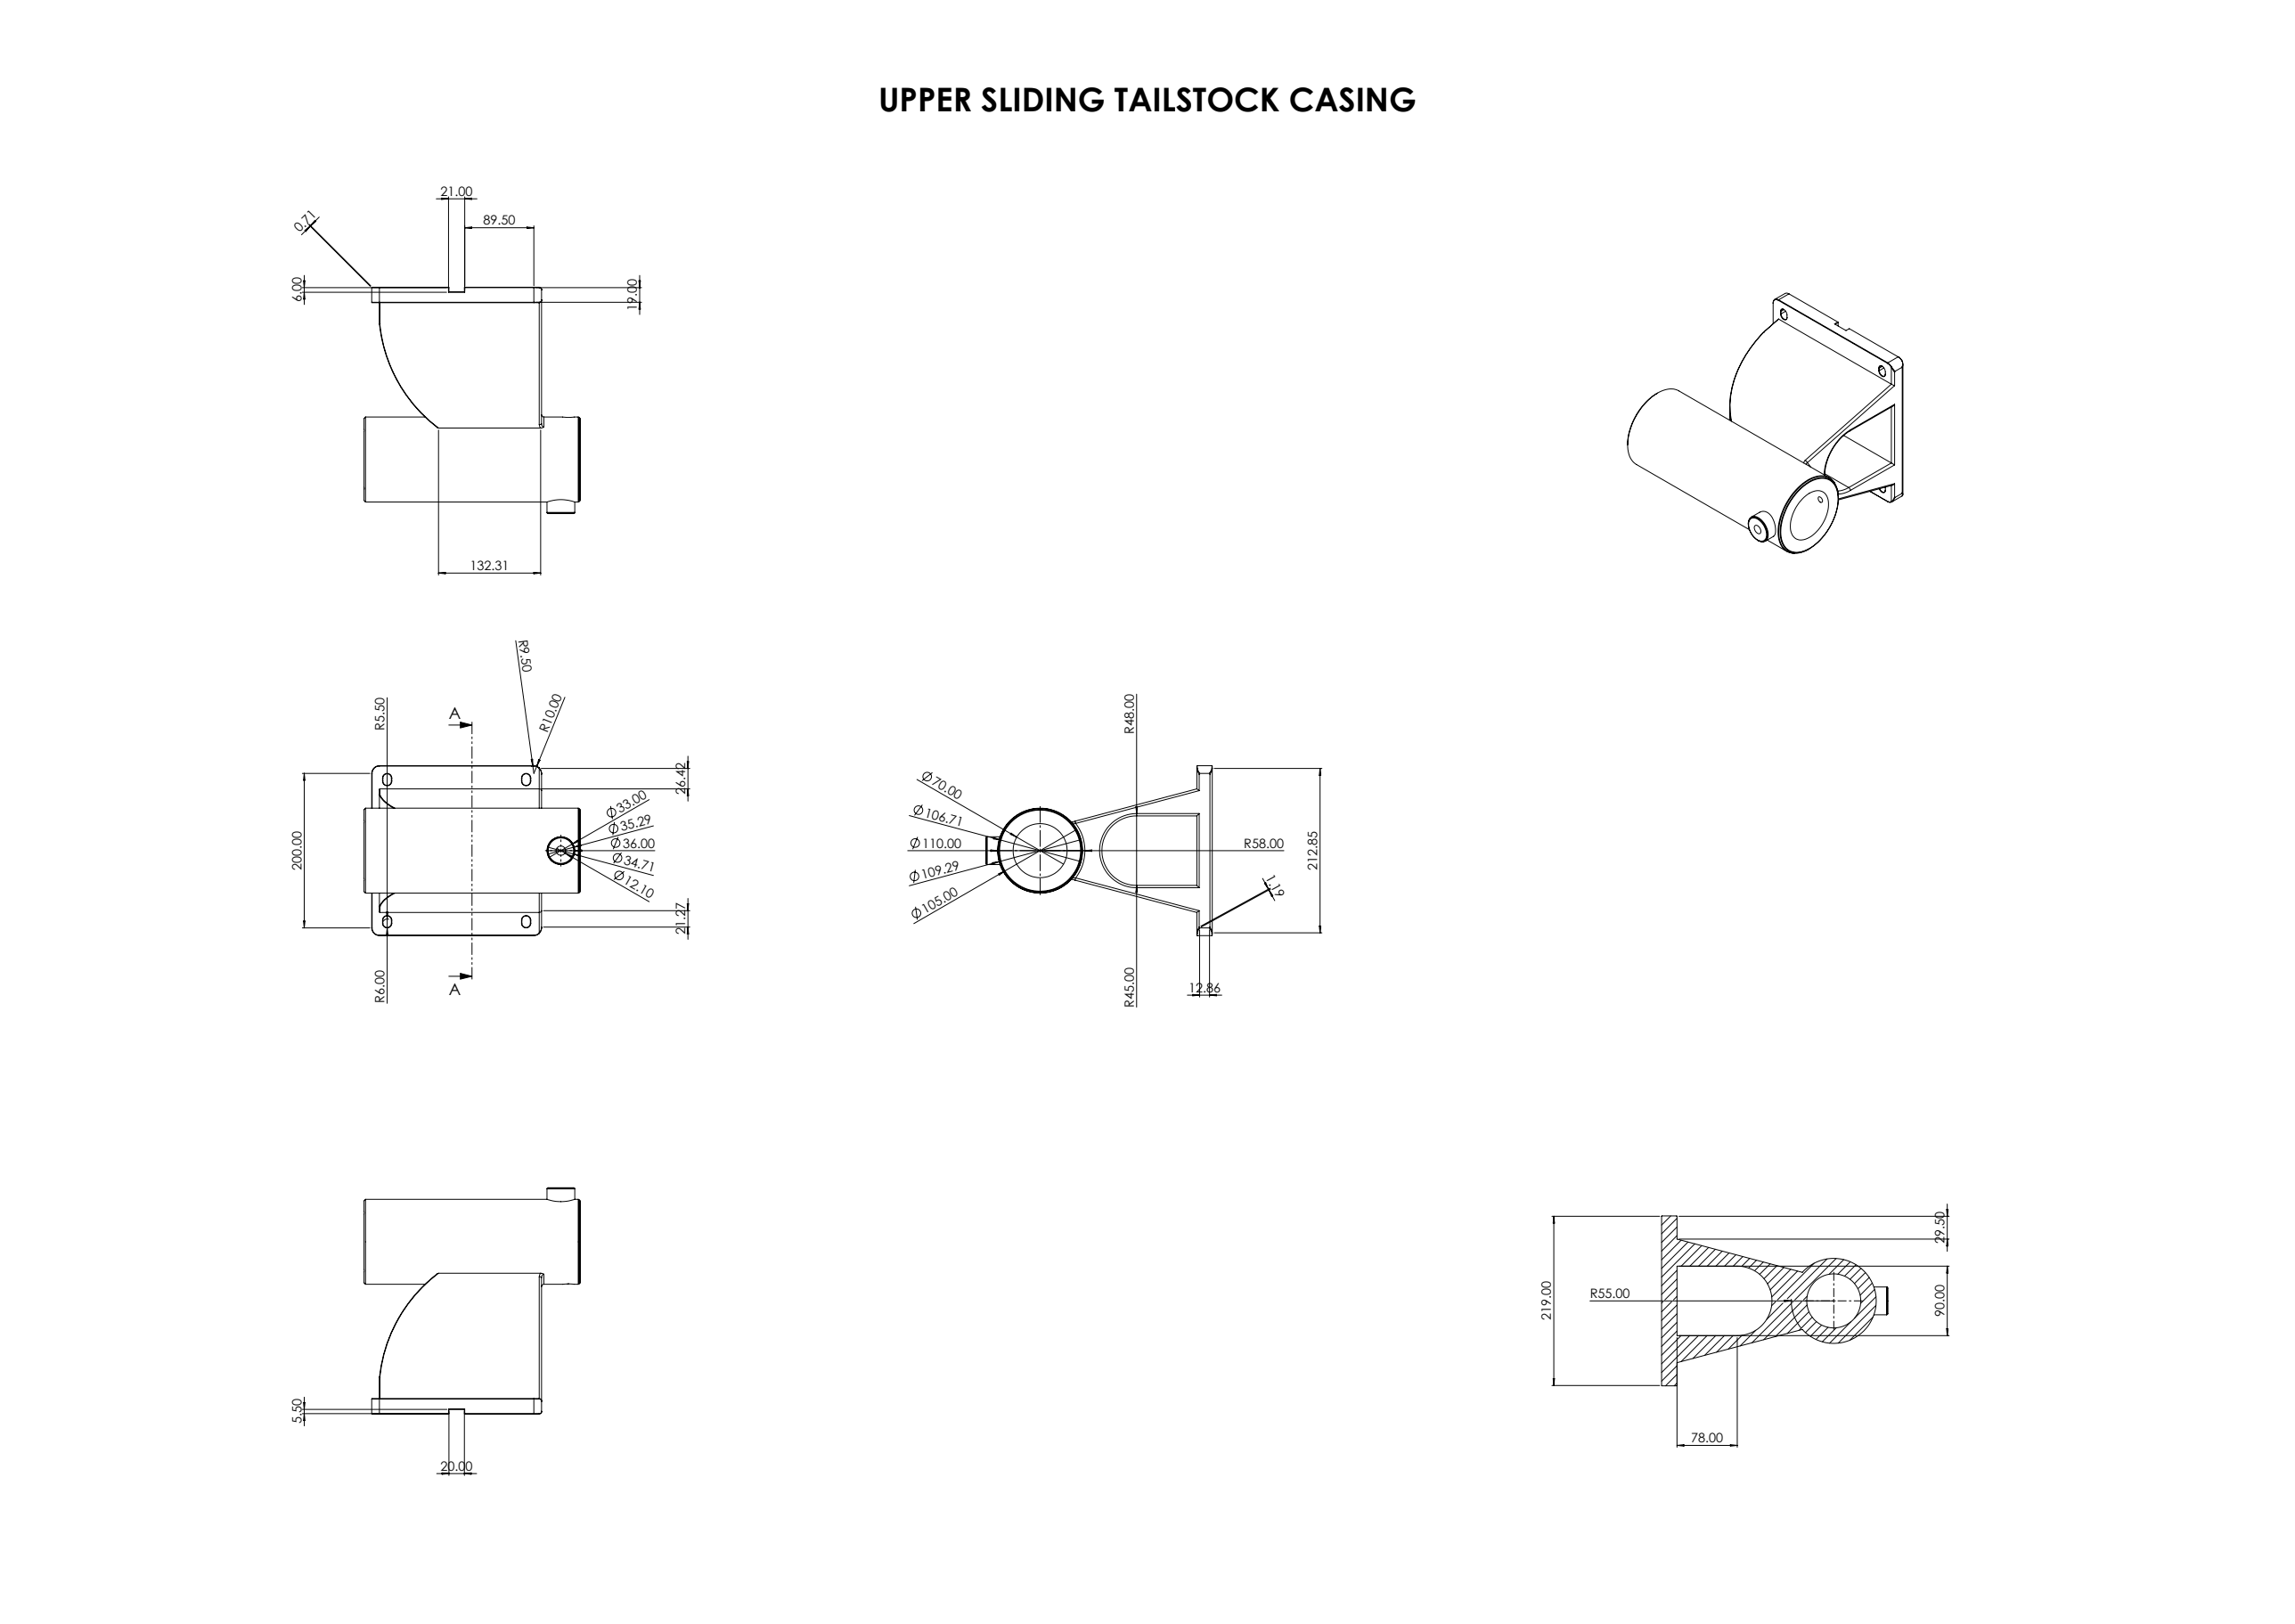
ISO-10303-21;
HEADER;
/* Generated by software containing ST-Developer
 * from STEP Tools, Inc. (www.steptools.com) 
 */

FILE_DESCRIPTION(
/* description */ (''),
/* implementation_level */ '2;1');

FILE_NAME(
/* name */ '02_Upper_Sliding_Tailstock_Casing.step',
/* time_stamp */ '2026-10-26T03:50:32-07:00',
/* author */ (''),
/* organization */ (''),
/* preprocessor_version */ 'ST-DEVELOPER v20.2',
/* originating_system */ 'Autodesk Translation Framework v15.15.0.0',
/* authorisation */ '');

FILE_SCHEMA (('AUTOMOTIVE_DESIGN { 1 0 10303 214 3 1 1 }'));
ENDSEC;

DATA;
#10=MECHANICAL_DESIGN_GEOMETRIC_PRESENTATION_REPRESENTATION('',(#1040),#76660);
#138=B_SPLINE_SURFACE_WITH_KNOTS('',3,3,((#37277,#37278,#37279,#37280,#37281,
#37282,#37283,#37284,#37285,#37286,#37287,#37288,#37289,#37290,#37291,#37292,
#37293,#37294,#37295,#37296,#37297,#37298,#37299,#37300,#37301,#37302,#37303,
#37304,#37305,#37306,#37307,#37308,#37309,#37310,#37311,#37312,#37313,#37314,
#37315,#37316,#37317,#37318,#37319,#37320,#37321,#37322,#37323,#37324),
(#37325,#37326,#37327,#37328,#37329,#37330,#37331,#37332,#37333,#37334,
#37335,#37336,#37337,#37338,#37339,#37340,#37341,#37342,#37343,#37344,#37345,
#37346,#37347,#37348,#37349,#37350,#37351,#37352,#37353,#37354,#37355,#37356,
#37357,#37358,#37359,#37360,#37361,#37362,#37363,#37364,#37365,#37366,#37367,
#37368,#37369,#37370,#37371,#37372),(#37373,#37374,#37375,#37376,#37377,
#37378,#37379,#37380,#37381,#37382,#37383,#37384,#37385,#37386,#37387,#37388,
#37389,#37390,#37391,#37392,#37393,#37394,#37395,#37396,#37397,#37398,#37399,
#37400,#37401,#37402,#37403,#37404,#37405,#37406,#37407,#37408,#37409,#37410,
#37411,#37412,#37413,#37414,#37415,#37416,#37417,#37418,#37419,#37420),
(#37421,#37422,#37423,#37424,#37425,#37426,#37427,#37428,#37429,#37430,
#37431,#37432,#37433,#37434,#37435,#37436,#37437,#37438,#37439,#37440,#37441,
#37442,#37443,#37444,#37445,#37446,#37447,#37448,#37449,#37450,#37451,#37452,
#37453,#37454,#37455,#37456,#37457,#37458,#37459,#37460,#37461,#37462,#37463,
#37464,#37465,#37466,#37467,#37468)),.UNSPECIFIED.,.F.,.T.,.F.,(4,4),(4,
1,1,1,1,1,1,1,1,1,1,1,1,1,1,1,1,1,1,1,1,1,1,1,1,1,1,1,1,1,1,1,1,1,1,1,1,
1,1,1,1,1,1,1,1,4),(0.,1.),(0.,0.301700924572155,0.452551386858232,0.60340184914431,
0.62225815693007,0.641114464715829,0.678827080287349,0.716539695858868,
0.754252311430387,0.829677542573426,0.867390158144946,0.905102773716465,
1.20680369828862,1.23194544200297,1.25708718571731,1.307370673146,1.40793764800339,
1.81020554743293,1.83534729114728,1.86048903486162,1.91077252229031,2.0113394971477,
2.21247344686247,2.26275693429116,2.41360739657724,2.56445785886332,2.71530832114939,
2.86615878343547,2.94158401457851,2.96044032236427,2.97929663015003,2.99815293793579,
3.00758109182867,3.01229516877511,3.01700924572155,3.3187101702937,3.35642278586522,
3.39413540143674,3.46956063257978,3.54498586372282,3.58269847929434,3.6015547870801,
3.62041109486586,3.77126155715194,3.92211201943801,4.22381294401017),
 .UNSPECIFIED.);
#139=B_SPLINE_SURFACE_WITH_KNOTS('',3,3,((#37678,#37679,#37680,#37681,#37682,
#37683,#37684,#37685),(#37686,#37687,#37688,#37689,#37690,#37691,#37692,
#37693),(#37694,#37695,#37696,#37697,#37698,#37699,#37700,#37701),(#37702,
#37703,#37704,#37705,#37706,#37707,#37708,#37709)),.UNSPECIFIED.,.F.,.F.,
 .F.,(4,4),(4,1,1,1,1,4),(0.,1.),(0.,0.142857142857143,0.428571428571429,
0.571428571428571,0.857142857142857,1.),.UNSPECIFIED.);
#140=B_SPLINE_SURFACE_WITH_KNOTS('',3,3,((#37811,#37812,#37813,#37814,#37815,
#37816,#37817,#37818),(#37819,#37820,#37821,#37822,#37823,#37824,#37825,
#37826),(#37827,#37828,#37829,#37830,#37831,#37832,#37833,#37834),(#37835,
#37836,#37837,#37838,#37839,#37840,#37841,#37842)),.UNSPECIFIED.,.F.,.F.,
 .F.,(4,4),(4,1,1,1,1,4),(0.,1.),(0.,0.142857142857143,0.428571428571429,
0.571428571428571,0.857142857142857,1.),.UNSPECIFIED.);
#141=B_SPLINE_SURFACE_WITH_KNOTS('',3,3,((#37944,#37945,#37946,#37947,#37948),
(#37949,#37950,#37951,#37952,#37953),(#37954,#37955,#37956,#37957,#37958),
(#37959,#37960,#37961,#37962,#37963)),.UNSPECIFIED.,.F.,.F.,.F.,(4,4),(4,
1,4),(0.,1.),(1.87779361595245,2.32640602317479,2.66286532859155),
 .UNSPECIFIED.);
#142=B_SPLINE_SURFACE_WITH_KNOTS('',3,3,((#38058,#38059,#38060,#38061),
(#38062,#38063,#38064,#38065),(#38066,#38067,#38068,#38069),(#38070,#38071,
#38072,#38073)),.UNSPECIFIED.,.F.,.F.,.F.,(4,4),(4,4),(0.,1.),(-1.87779361595245,
-1.82480525135948),.UNSPECIFIED.);
#143=B_SPLINE_SURFACE_WITH_KNOTS('',3,3,((#38078,#38079,#38080,#38081,#38082),
(#38083,#38084,#38085,#38086,#38087),(#38088,#38089,#38090,#38091,#38092),
(#38093,#38094,#38095,#38096,#38097)),.UNSPECIFIED.,.F.,.F.,.F.,(4,4),(4,
1,4),(0.,1.),(0.000100035134689748,0.3365592783323,0.78517160259578),
 .UNSPECIFIED.);
#144=B_SPLINE_SURFACE_WITH_KNOTS('',3,3,((#38110,#38111,#38112,#38113),
(#38114,#38115,#38116,#38117),(#38118,#38119,#38120,#38121),(#38122,#38123,
#38124,#38125)),.UNSPECIFIED.,.F.,.F.,.F.,(4,4),(4,4),(0.,1.),(-0.838159967188763,
-0.78517160259578),.UNSPECIFIED.);
#145=B_SPLINE_SURFACE_WITH_KNOTS('',3,3,((#38503,#38504,#38505,#38506,#38507,
#38508,#38509,#38510),(#38511,#38512,#38513,#38514,#38515,#38516,#38517,
#38518),(#38519,#38520,#38521,#38522,#38523,#38524,#38525,#38526),(#38527,
#38528,#38529,#38530,#38531,#38532,#38533,#38534)),.UNSPECIFIED.,.F.,.F.,
 .F.,(4,4),(4,1,1,1,1,4),(0.,1.),(0.,0.142857142857143,0.428571428571429,
0.571428571428571,0.857142857142857,1.),.UNSPECIFIED.);
#146=B_SPLINE_SURFACE_WITH_KNOTS('',3,3,((#38592,#38593,#38594,#38595,#38596,
#38597,#38598,#38599),(#38600,#38601,#38602,#38603,#38604,#38605,#38606,
#38607),(#38608,#38609,#38610,#38611,#38612,#38613,#38614,#38615),(#38616,
#38617,#38618,#38619,#38620,#38621,#38622,#38623)),.UNSPECIFIED.,.F.,.F.,
 .F.,(4,4),(4,1,1,1,1,4),(0.,1.),(0.,0.142857142857143,0.428571428571429,
0.571428571428571,0.857142857142857,1.),.UNSPECIFIED.);
#147=B_SPLINE_SURFACE_WITH_KNOTS('',3,3,((#38722,#38723,#38724,#38725,#38726,
#38727,#38728),(#38729,#38730,#38731,#38732,#38733,#38734,#38735),(#38736,
#38737,#38738,#38739,#38740,#38741,#38742),(#38743,#38744,#38745,#38746,
#38747,#38748,#38749)),.UNSPECIFIED.,.F.,.F.,.F.,(4,4),(4,1,1,1,4),(0.,
1.),(9.97415695384386E-5,0.217192720402113,0.325739209818401,0.542832188650975,
0.75992516748355),.UNSPECIFIED.);
#148=B_SPLINE_SURFACE_WITH_KNOTS('',3,3,((#38791,#38792,#38793,#38794),
(#38795,#38796,#38797,#38798),(#38799,#38800,#38801,#38802),(#38803,#38804,
#38805,#38806)),.UNSPECIFIED.,.F.,.F.,.F.,(4,4),(4,4),(0.,1.),(0.759925167483548,
0.811761172549836),.UNSPECIFIED.);
#149=B_SPLINE_SURFACE_WITH_KNOTS('',3,3,((#38811,#38812,#38813,#38814,#38815,
#38816,#38817,#38818,#38819,#38820),(#38821,#38822,#38823,#38824,#38825,
#38826,#38827,#38828,#38829,#38830),(#38831,#38832,#38833,#38834,#38835,
#38836,#38837,#38838,#38839,#38840),(#38841,#38842,#38843,#38844,#38845,
#38846,#38847,#38848,#38849,#38850)),.UNSPECIFIED.,.F.,.F.,.F.,(4,4),(4,
2,1,1,2,4),(0.,1.),(1.90304005106469,2.0340806772701,2.19643291178007,2.27760902903505,
2.43996126354502,2.66286552223545),.UNSPECIFIED.);
#150=B_SPLINE_SURFACE_WITH_KNOTS('',3,3,((#38862,#38863,#38864,#38865),
(#38866,#38867,#38868,#38869),(#38870,#38871,#38872,#38873),(#38874,#38875,
#38876,#38877)),.UNSPECIFIED.,.F.,.F.,.F.,(4,4),(4,4),(0.,1.),(1.85120404599841,
1.90304005106469),.UNSPECIFIED.);
#151=B_SPLINE_SURFACE_WITH_KNOTS('',3,3,((#38903,#38904,#38905,#38906,#38907,
#38908,#38909,#38910,#38911,#38912,#38913,#38914,#38915,#38916,#38917,#38918,
#38919,#38920,#38921,#38922),(#38923,#38924,#38925,#38926,#38927,#38928,
#38929,#38930,#38931,#38932,#38933,#38934,#38935,#38936,#38937,#38938,#38939,
#38940,#38941,#38942),(#38943,#38944,#38945,#38946,#38947,#38948,#38949,
#38950,#38951,#38952,#38953,#38954,#38955,#38956,#38957,#38958,#38959,#38960,
#38961,#38962),(#38963,#38964,#38965,#38966,#38967,#38968,#38969,#38970,
#38971,#38972,#38973,#38974,#38975,#38976,#38977,#38978,#38979,#38980,#38981,
#38982)),.UNSPECIFIED.,.F.,.F.,.F.,(4,4),(4,1,1,1,1,1,1,1,1,1,1,1,1,1,1,
1,1,4),(0.,1.),(6.93617595249389,7.96866100733354,9.0011460621732,10.0336311170129,
10.5498736444327,11.0661161718525,12.0986012266922,13.1310862815318,13.8194096514249,
14.507733021318,15.1960563912111,16.5727031309973,17.2610265008905,17.7772690283103,
18.2935115557301,19.3259966105698,20.3584816654094,21.3909667202491),
 .UNSPECIFIED.);
#152=B_SPLINE_SURFACE_WITH_KNOTS('',3,3,((#39029,#39030,#39031,#39032),
(#39033,#39034,#39035,#39036),(#39037,#39038,#39039,#39040),(#39041,#39042,
#39043,#39044)),.UNSPECIFIED.,.F.,.F.,.F.,(4,4),(4,4),(0.,1.),(6.91671820418794,
6.93617595249389),.UNSPECIFIED.);
#153=B_SPLINE_SURFACE_WITH_KNOTS('',3,3,((#39053,#39054,#39055,#39056),
(#39057,#39058,#39059,#39060),(#39061,#39062,#39063,#39064),(#39065,#39066,
#39067,#39068)),.UNSPECIFIED.,.F.,.F.,.F.,(4,4),(4,4),(0.,1.),(21.3909667202491,
21.410424468555),.UNSPECIFIED.);
#154=B_SPLINE_SURFACE_WITH_KNOTS('',3,3,((#39101,#39102,#39103,#39104,#39105,
#39106,#39107),(#39108,#39109,#39110,#39111,#39112,#39113,#39114),(#39115,
#39116,#39117,#39118,#39119,#39120,#39121),(#39122,#39123,#39124,#39125,
#39126,#39127,#39128)),.UNSPECIFIED.,.F.,.F.,.F.,(4,4),(4,1,1,1,4),(0.,
1.),(0.645522939086389,0.821861702311259,0.998200465536129,1.23331881650262,
1.46843716746911),.UNSPECIFIED.);
#155=B_SPLINE_SURFACE_WITH_KNOTS('',3,3,((#39165,#39166,#39167,#39168,#39169,
#39170,#39171),(#39172,#39173,#39174,#39175,#39176,#39177,#39178),(#39179,
#39180,#39181,#39182,#39183,#39184,#39185),(#39186,#39187,#39188,#39189,
#39190,#39191,#39192)),.UNSPECIFIED.,.F.,.F.,.F.,(4,4),(4,1,1,1,4),(0.,
1.),(-1.46843716746912,-1.29209840424425,-1.11575964101938,-0.880641290052883,
-0.645522939086389),.UNSPECIFIED.);
#156=B_SPLINE_SURFACE_WITH_KNOTS('',3,3,((#39211,#39212,#39213,#39214,#39215,
#39216),(#39217,#39218,#39219,#39220,#39221,#39222),(#39223,#39224,#39225,
#39226,#39227,#39228),(#39229,#39230,#39231,#39232,#39233,#39234),(#39235,
#39236,#39237,#39238,#39239,#39240)),.UNSPECIFIED.,.F.,.F.,.F.,(4,1,4),
(4,1,1,4),(0.,0.571428571428571,1.),(3.93038111840777,4.35323723299001,
4.63514130937817,4.91704538576632),.UNSPECIFIED.);
#157=B_SPLINE_SURFACE_WITH_KNOTS('',3,3,((#39269,#39270,#39271,#39272,#39273,
#39274),(#39275,#39276,#39277,#39278,#39279,#39280),(#39281,#39282,#39283,
#39284,#39285,#39286),(#39287,#39288,#39289,#39290,#39291,#39292),(#39293,
#39294,#39295,#39296,#39297,#39298)),.UNSPECIFIED.,.F.,.F.,.F.,(4,1,4),
(4,1,1,4),(0.,0.571428571428571,1.),(0.317698823900363,0.599602900914624,
0.740554939421754,1.30436309345028),.UNSPECIFIED.);
#174=B_SPLINE_CURVE_WITH_KNOTS('',3,(#37067,#37068,#37069,#37070,#37071,
#37072,#37073,#37074,#37075,#37076,#37077,#37078,#37079,#37080,#37081,#37082,
#37083,#37084),.UNSPECIFIED.,.F.,.F.,(4,2,2,2,2,2,2,2,4),(0.,0.341830025609023,
0.683660051218047,1.02549007682707,1.36732010243609,1.7090034027405,2.05068670304491,
2.39237000334931,2.73405330365372),.UNSPECIFIED.);
#175=B_SPLINE_CURVE_WITH_KNOTS('',3,(#37085,#37086,#37087,#37088,#37089,
#37090,#37091,#37092,#37093,#37094,#37095,#37096,#37097,#37098,#37099,#37100,
#37101,#37102,#37103,#37104,#37105,#37106,#37107,#37108,#37109,#37110,#37111,
#37112,#37113,#37114,#37115,#37116,#37117,#37118,#37119,#37120,#37121,#37122,
#37123,#37124,#37125,#37126,#37127,#37128,#37129,#37130,#37131,#37132,#37133,
#37134),.UNSPECIFIED.,.F.,.F.,(4,2,2,2,2,2,2,2,2,2,2,2,2,2,2,2,2,2,2,2,
2,2,2,2,4),(2.73405330365372,3.07573660395812,3.41741990426253,3.75910320456694,
4.10078650487134,4.44261653048037,4.78444655608939,5.12627658169841,5.46810660730744,
5.80993663291646,6.15176665852548,6.49359668413451,6.83542670974353,7.17711001004794,
7.51879331035234,7.86047661065675,8.20215991096115,8.54384321126556,8.88552651156997,
9.22720981187437,9.56889311217878,9.9107231377878,10.2525531633968,10.5943831890058,
10.9362132146149),.UNSPECIFIED.);
#176=B_SPLINE_CURVE_WITH_KNOTS('',3,(#37138,#37139,#37140,#37141,#37142,
#37143),.UNSPECIFIED.,.F.,.F.,(4,2,4),(1.71566353344894,1.90989804259815,
2.10413255174736),.UNSPECIFIED.);
#177=B_SPLINE_CURVE_WITH_KNOTS('',3,(#37163,#37164,#37165,#37166,#37167,
#37168),.UNSPECIFIED.,.F.,.F.,(4,2,4),(1.71566348905116,1.90989799807537,
2.10413250709959),.UNSPECIFIED.);
#178=B_SPLINE_CURVE_WITH_KNOTS('',3,(#37172,#37173,#37174,#37175,#37176,
#37177),.UNSPECIFIED.,.F.,.F.,(4,2,4),(1.71529227392093,1.90952573777923,
2.10375920163752),.UNSPECIFIED.);
#179=B_SPLINE_CURVE_WITH_KNOTS('',3,(#37181,#37182,#37183,#37184,#37185,
#37186),.UNSPECIFIED.,.F.,.F.,(4,2,4),(1.7156635334436,1.90989804259278,
2.10413255174196),.UNSPECIFIED.);
#180=B_SPLINE_CURVE_WITH_KNOTS('',3,(#37222,#37223,#37224,#37225),
 .UNSPECIFIED.,.F.,.F.,(4,4),(-1.87779361595245,-1.82480525135948),
 .UNSPECIFIED.);
#181=B_SPLINE_CURVE_WITH_KNOTS('',3,(#37229,#37230,#37231,#37232),
 .UNSPECIFIED.,.F.,.F.,(4,4),(-0.838159967188763,-0.78517160259578),
 .UNSPECIFIED.);
#182=B_SPLINE_CURVE_WITH_KNOTS('',3,(#37473,#37474,#37475,#37476,#37477,
#37478,#37479,#37480,#37481,#37482,#37483,#37484,#37485,#37486,#37487,#37488,
#37489,#37490,#37491,#37492,#37493,#37494,#37495,#37496,#37497,#37498,#37499,
#37500,#37501,#37502,#37503,#37504,#37505,#37506,#37507,#37508,#37509,#37510),
 .UNSPECIFIED.,.F.,.F.,(4,1,1,1,1,1,1,1,1,1,1,1,1,1,1,1,1,1,1,1,1,1,1,1,
1,1,1,1,1,1,1,1,1,1,1,4),(0.,0.301700924572155,0.452551386858232,0.60340184914431,
0.62225815693007,0.641114464715829,0.678827080287349,0.716539695858868,
0.754252311430387,0.829677542573426,0.867390158144946,0.905102773716465,
1.20680369828862,1.23194544200297,1.25708718571731,1.307370673146,1.40793764800339,
1.81020554743293,1.83534729114728,1.86048903486162,1.91077252229031,2.0113394971477,
2.21247344686247,2.26275693429116,2.41360739657724,2.56445785886332,2.71530832114939,
2.86615878343547,2.94158401457851,2.96044032236427,2.97929663015003,2.99815293793579,
3.00758109182867,3.01229516877511,3.01700924572155,3.16785970800763),
 .UNSPECIFIED.);
#183=B_SPLINE_CURVE_WITH_KNOTS('',3,(#37511,#37512,#37513,#37514,#37515,
#37516,#37517,#37518,#37519,#37520,#37521,#37522,#37523,#37524),
 .UNSPECIFIED.,.F.,.F.,(4,1,1,1,1,1,1,1,1,1,1,4),(3.16785970800763,3.3187101702937,
3.35642278586522,3.39413540143674,3.46956063257978,3.54498586372282,3.58269847929434,
3.6015547870801,3.62041109486586,3.77126155715194,3.92211201943801,4.22381294401017),
 .UNSPECIFIED.);
#184=B_SPLINE_CURVE_WITH_KNOTS('',3,(#37525,#37526,#37527,#37528,#37529,
#37530,#37531,#37532,#37533,#37534,#37535,#37536,#37537,#37538,#37539,#37540,
#37541,#37542,#37543,#37544,#37545,#37546,#37547,#37548,#37549,#37550,#37551,
#37552,#37553,#37554,#37555,#37556,#37557,#37558,#37559,#37560,#37561,#37562,
#37563,#37564,#37565,#37566,#37567,#37568,#37569,#37570,#37571,#37572),
 .UNSPECIFIED.,.T.,.F.,(4,1,1,1,1,1,1,1,1,1,1,1,1,1,1,1,1,1,1,1,1,1,1,1,
1,1,1,1,1,1,1,1,1,1,1,1,1,1,1,1,1,1,1,1,1,4),(-4.22381294401017,-3.92211201943801,
-3.77126155715194,-3.62041109486586,-3.6015547870801,-3.58269847929434,
-3.54498586372282,-3.46956063257978,-3.39413540143674,-3.35642278586522,
-3.3187101702937,-3.01700924572155,-3.01229516877511,-3.00758109182867,
-2.99815293793579,-2.97929663015003,-2.96044032236427,-2.94158401457851,
-2.86615878343547,-2.71530832114939,-2.56445785886332,-2.41360739657724,
-2.26275693429116,-2.21247344686247,-2.0113394971477,-1.91077252229031,
-1.86048903486162,-1.83534729114728,-1.81020554743293,-1.40793764800339,
-1.307370673146,-1.25708718571731,-1.23194544200297,-1.20680369828862,-0.905102773716465,
-0.867390158144946,-0.829677542573426,-0.754252311430387,-0.716539695858868,
-0.678827080287349,-0.641114464715829,-0.62225815693007,-0.60340184914431,
-0.452551386858232,-0.301700924572155,0.),.UNSPECIFIED.);
#185=B_SPLINE_CURVE_WITH_KNOTS('',3,(#37583,#37584,#37585,#37586,#37587,
#37588,#37589),.UNSPECIFIED.,.F.,.F.,(4,3,4),(0.,0.0706076080518625,0.140717785645037),
 .UNSPECIFIED.);
#186=B_SPLINE_CURVE_WITH_KNOTS('',3,(#37591,#37592,#37593,#37594,#37595,
#37596,#37597,#37598,#37599,#37600,#37601,#37602,#37603,#37604,#37605,#37606,
#37607,#37608,#37609,#37610,#37611,#37612,#37613,#37614,#37615,#37616,#37617),
 .UNSPECIFIED.,.F.,.F.,(4,2,2,2,2,2,3,2,2,2,2,2,4),(-4.20812861828807,-3.99425066999856,
-3.16073871853832,-2.37055403890373,-1.58036935926916,-0.790184679634578,
0.,0.79018467963458,1.58036935926916,2.37055403890374,3.16073871853832,
3.99425066999856,4.20812861828807),.UNSPECIFIED.);
#187=B_SPLINE_CURVE_WITH_KNOTS('',3,(#37619,#37620,#37621,#37622,#37623,
#37624,#37625),.UNSPECIFIED.,.F.,.F.,(4,3,4),(0.,0.0701050024887815,0.140717775218191),
 .UNSPECIFIED.);
#188=B_SPLINE_CURVE_WITH_KNOTS('',3,(#37629,#37630,#37631,#37632,#37633,
#37634,#37635,#37636,#37637,#37638),.UNSPECIFIED.,.F.,.F.,(4,2,2,2,4),(0.,
0.120853732558559,0.299961593709033,0.490853831409324,0.492261507196457),
 .UNSPECIFIED.);
#189=B_SPLINE_CURVE_WITH_KNOTS('',3,(#37641,#37642,#37643,#37644,#37645,
#37646,#37647,#37648,#37649,#37650),.UNSPECIFIED.,.F.,.F.,(4,2,2,2,4),(-0.00109523829507863,
0.,0.141893095426123,0.28665904951154,0.476004129030812),.UNSPECIFIED.);
#190=B_SPLINE_CURVE_WITH_KNOTS('',3,(#37712,#37713,#37714,#37715,#37716,
#37717,#37718,#37719,#37720,#37721,#37722,#37723,#37724,#37725,#37726,#37727,
#37728,#37729,#37730,#37731,#37732,#37733,#37734,#37735,#37736,#37737,#37738,
#37739,#37740,#37741,#37742,#37743,#37744,#37745,#37746,#37747,#37748,#37749,
#37750,#37751),.UNSPECIFIED.,.F.,.F.,(4,3,3,3,3,3,3,3,3,3,3,3,3,4),(0.,
0.0642058267314402,0.135298039610793,0.216720613163576,0.322214526794598,
0.406937710945273,0.476869411739625,0.550300205763178,0.627974002306146,
0.731399879303705,0.815726896068677,0.88866362574166,0.953773893187292,
1.),.UNSPECIFIED.);
#191=B_SPLINE_CURVE_WITH_KNOTS('',3,(#37753,#37754,#37755,#37756),
 .UNSPECIFIED.,.F.,.F.,(4,4),(0.,1.),.UNSPECIFIED.);
#192=B_SPLINE_CURVE_WITH_KNOTS('',3,(#37758,#37759,#37760,#37761,#37762,
#37763,#37764,#37765,#37766,#37767,#37768,#37769,#37770,#37771,#37772,#37773,
#37774,#37775,#37776,#37777,#37778,#37779,#37780,#37781,#37782,#37783,#37784,
#37785,#37786,#37787,#37788,#37789,#37790,#37791,#37792,#37793,#37794,#37795,
#37796,#37797,#37798,#37799,#37800,#37801,#37802,#37803,#37804,#37805,#37806,
#37807,#37808,#37809),.UNSPECIFIED.,.F.,.F.,(4,3,3,3,3,3,3,3,3,3,3,3,3,
3,3,3,3,4),(0.,0.0470013637169586,0.0964181016740628,0.149229530335118,
0.208169836206556,0.286934368114381,0.357340819180099,0.414362060111408,
0.466217667030896,0.532940458652034,0.585846875133388,0.644811876239638,
0.72711087277581,0.795333154581857,0.850882587463839,0.902663377962928,
0.951331688981464,1.),.UNSPECIFIED.);
#193=B_SPLINE_CURVE_WITH_KNOTS('',3,(#37845,#37846,#37847,#37848,#37849,
#37850,#37851,#37852,#37853,#37854,#37855,#37856,#37857,#37858,#37859,#37860,
#37861,#37862,#37863,#37864,#37865,#37866,#37867,#37868,#37869,#37870,#37871,
#37872,#37873,#37874,#37875,#37876,#37877,#37878,#37879,#37880,#37881,#37882,
#37883,#37884,#37885,#37886,#37887,#37888,#37889,#37890,#37891,#37892,#37893,
#37894,#37895,#37896),.UNSPECIFIED.,.F.,.F.,(4,3,3,3,3,3,3,3,3,3,3,3,3,
3,3,3,3,4),(0.,0.0469954003122149,0.0964054107400102,0.149208793967372,
0.208136804390094,0.286850662832856,0.357279255948468,0.414301991680454,
0.466156507957792,0.532886944463068,0.585793820692173,0.644755325044784,
0.727049300721868,0.795286975541401,0.85084796357777,0.9026376409811,0.95131882049055,
1.),.UNSPECIFIED.);
#194=B_SPLINE_CURVE_WITH_KNOTS('',3,(#37898,#37899,#37900,#37901),
 .UNSPECIFIED.,.F.,.F.,(4,4),(-1.,0.),.UNSPECIFIED.);
#195=B_SPLINE_CURVE_WITH_KNOTS('',3,(#37903,#37904,#37905,#37906,#37907,
#37908,#37909,#37910,#37911,#37912,#37913,#37914,#37915,#37916,#37917,#37918,
#37919,#37920,#37921,#37922,#37923,#37924,#37925,#37926,#37927,#37928,#37929,
#37930,#37931,#37932,#37933,#37934,#37935,#37936,#37937,#37938,#37939,#37940,
#37941,#37942),.UNSPECIFIED.,.F.,.F.,(4,3,3,3,3,3,3,3,3,3,3,3,3,4),(0.,
0.0642045803508197,0.135295214744166,0.216715461741643,0.322211745001425,
0.406935276876247,0.476866299954066,0.550298370624421,0.62797200200528,
0.73139484549015,0.815724459936111,0.888662483366991,0.953773603714735,
1.),.UNSPECIFIED.);
#196=B_SPLINE_CURVE_WITH_KNOTS('',3,(#37964,#37965,#37966,#37967,#37968),
 .UNSPECIFIED.,.F.,.F.,(4,1,4),(-2.66286532859155,-2.32640602317479,-1.87779361595245),
 .UNSPECIFIED.);
#197=B_SPLINE_CURVE_WITH_KNOTS('',3,(#37971,#37972,#37973,#37974,#37975),
 .UNSPECIFIED.,.F.,.F.,(4,1,4),(1.87779361595245,2.32640602317479,2.66286532859155),
 .UNSPECIFIED.);
#198=B_SPLINE_CURVE_WITH_KNOTS('',3,(#38074,#38075,#38076,#38077),
 .UNSPECIFIED.,.F.,.F.,(4,4),(1.82480525135948,1.87779361595245),
 .UNSPECIFIED.);
#199=B_SPLINE_CURVE_WITH_KNOTS('',3,(#38099,#38100,#38101,#38102,#38103),
 .UNSPECIFIED.,.F.,.F.,(4,1,4),(0.000100035134689748,0.3365592783323,0.78517160259578),
 .UNSPECIFIED.);
#200=B_SPLINE_CURVE_WITH_KNOTS('',3,(#38105,#38106,#38107,#38108,#38109),
 .UNSPECIFIED.,.F.,.F.,(4,1,4),(-0.78517160259578,-0.3365592783323,-0.000100035134689748),
 .UNSPECIFIED.);
#201=B_SPLINE_CURVE_WITH_KNOTS('',3,(#38126,#38127,#38128,#38129),
 .UNSPECIFIED.,.F.,.F.,(4,4),(0.78517160259578,0.838159967188763),
 .UNSPECIFIED.);
#202=B_SPLINE_CURVE_WITH_KNOTS('',3,(#38140,#38141,#38142,#38143,#38144,
#38145,#38146,#38147,#38148,#38149,#38150,#38151,#38152,#38153,#38154,#38155,
#38156,#38157,#38158,#38159,#38160,#38161,#38162,#38163,#38164,#38165,#38166,
#38167,#38168,#38169,#38170,#38171,#38172,#38173,#38174,#38175,#38176,#38177,
#38178,#38179),.UNSPECIFIED.,.F.,.F.,(4,3,3,3,3,3,3,3,3,3,3,3,3,4),(0.,
0.0642049615968745,0.13529611806662,0.216717311062181,0.322210830481009,
0.406934476670883,0.476865564838168,0.550296903893395,0.627969426873969,
0.73138741425766,0.815717741324156,0.888655709551853,0.95376643384809,1.),
 .UNSPECIFIED.);
#203=B_SPLINE_CURVE_WITH_KNOTS('',3,(#38181,#38182,#38183,#38184,#38185,
#38186,#38187,#38188,#38189,#38190),.UNSPECIFIED.,.F.,.F.,(4,2,1,1,2,4),
(1.90304005106469,2.0340806772701,2.19643291178007,2.27760902903505,2.43996126354502,
2.66286552223545),.UNSPECIFIED.);
#204=B_SPLINE_CURVE_WITH_KNOTS('',3,(#38192,#38193,#38194,#38195),
 .UNSPECIFIED.,.F.,.F.,(4,4),(1.85120404599841,1.90304005106469),
 .UNSPECIFIED.);
#205=B_SPLINE_CURVE_WITH_KNOTS('',3,(#38397,#38398,#38399,#38400),
 .UNSPECIFIED.,.F.,.F.,(4,4),(-1.90304005106469,-1.85120404599841),
 .UNSPECIFIED.);
#206=B_SPLINE_CURVE_WITH_KNOTS('',3,(#38423,#38424,#38425,#38426),
 .UNSPECIFIED.,.F.,.F.,(4,4),(-0.811761172549836,-0.759925167483548),
 .UNSPECIFIED.);
#207=B_SPLINE_CURVE_WITH_KNOTS('',3,(#38536,#38537,#38538,#38539,#38540,
#38541,#38542,#38543,#38544,#38545,#38546,#38547,#38548,#38549,#38550,#38551,
#38552,#38553,#38554,#38555,#38556,#38557,#38558,#38559,#38560,#38561,#38562,
#38563,#38564,#38565,#38566,#38567,#38568,#38569,#38570,#38571,#38572,#38573,
#38574,#38575,#38576,#38577,#38578,#38579,#38580,#38581,#38582,#38583,#38584,
#38585,#38586,#38587),.UNSPECIFIED.,.F.,.F.,(4,3,3,3,3,3,3,3,3,3,3,3,3,
3,3,3,3,4),(0.,0.0469948696945841,0.0964043092295198,0.149207058425544,
0.208134234796173,0.28684591375033,0.357274586919083,0.414296923289968,
0.466151007737128,0.532882131769987,0.585788839820251,0.644749528487852,
0.727041946185393,0.795281459639045,0.850844102970669,0.902635002958616,
0.951317501479308,1.),.UNSPECIFIED.);
#208=B_SPLINE_CURVE_WITH_KNOTS('',3,(#38588,#38589,#38590,#38591),
 .UNSPECIFIED.,.F.,.F.,(4,4),(-1.,0.),.UNSPECIFIED.);
#209=B_SPLINE_CURVE_WITH_KNOTS('',3,(#38625,#38626,#38627,#38628,#38629,
#38630,#38631,#38632,#38633,#38634,#38635,#38636,#38637,#38638,#38639,#38640,
#38641,#38642,#38643,#38644,#38645,#38646,#38647,#38648,#38649,#38650,#38651,
#38652,#38653,#38654,#38655,#38656,#38657,#38658,#38659,#38660,#38661,#38662,
#38663,#38664),.UNSPECIFIED.,.F.,.F.,(4,3,3,3,3,3,3,3,3,3,3,3,3,4),(0.,
0.0642044939750475,0.135295066626768,0.216715381562263,0.322209970902435,
0.406933724539631,0.476864590196812,0.550296651109942,0.627969500567193,
0.731388236611723,0.815719035368179,0.888657375631424,0.953768460302656,
1.),.UNSPECIFIED.);
#210=B_SPLINE_CURVE_WITH_KNOTS('',3,(#38666,#38667,#38668,#38669),
 .UNSPECIFIED.,.F.,.F.,(4,4),(0.,1.),.UNSPECIFIED.);
#211=B_SPLINE_CURVE_WITH_KNOTS('',3,(#38670,#38671,#38672,#38673,#38674,
#38675,#38676,#38677,#38678,#38679,#38680,#38681,#38682,#38683,#38684,#38685,
#38686,#38687,#38688,#38689,#38690,#38691,#38692,#38693,#38694,#38695,#38696,
#38697,#38698,#38699,#38700,#38701,#38702,#38703,#38704,#38705,#38706,#38707,
#38708,#38709,#38710,#38711,#38712,#38713,#38714,#38715,#38716,#38717,#38718,
#38719,#38720,#38721),.UNSPECIFIED.,.F.,.F.,(4,3,3,3,3,3,3,3,3,3,3,3,3,
3,3,3,3,4),(0.,0.0470027094723439,0.0964210394547843,0.149234501608351,
0.208178283267004,0.286960064846777,0.357356255023185,0.414375729071717,
0.466230636148304,0.532951806629766,0.585857475727138,0.644822009403465,
0.727120616369207,0.795340462276906,0.850888128017495,0.90266743730169,
0.951333718650845,1.),.UNSPECIFIED.);
#212=B_SPLINE_CURVE_WITH_KNOTS('',3,(#38751,#38752,#38753,#38754,#38755,
#38756,#38757),.UNSPECIFIED.,.F.,.F.,(4,1,1,1,4),(9.97415695384386E-5,0.217192720402113,
0.325739209818401,0.542832188650975,0.75992516748355),.UNSPECIFIED.);
#213=B_SPLINE_CURVE_WITH_KNOTS('',3,(#38759,#38760,#38761,#38762,#38763,
#38764,#38765),.UNSPECIFIED.,.F.,.F.,(4,1,1,1,4),(-0.75992516748355,-0.542832188650975,
-0.325739209818401,-0.217192720402113,-9.97415695384386E-5),
 .UNSPECIFIED.);
#214=B_SPLINE_CURVE_WITH_KNOTS('',3,(#38807,#38808,#38809,#38810),
 .UNSPECIFIED.,.F.,.F.,(4,4),(0.759925167483548,0.811761172549836),
 .UNSPECIFIED.);
#215=B_SPLINE_CURVE_WITH_KNOTS('',3,(#38851,#38852,#38853,#38854,#38855,
#38856,#38857,#38858,#38859,#38860),.UNSPECIFIED.,.F.,.F.,(4,2,1,1,2,4),
(-2.66286552223545,-2.43996126354502,-2.27760902903505,-2.19643291178007,
-2.0340806772701,-1.90304005106469),.UNSPECIFIED.);
#216=B_SPLINE_CURVE_WITH_KNOTS('',3,(#38893,#38894,#38895,#38896),
 .UNSPECIFIED.,.F.,.F.,(4,4),(0.,0.0707569587600326),.UNSPECIFIED.);
#217=B_SPLINE_CURVE_WITH_KNOTS('',3,(#38987,#38988,#38989,#38990,#38991,
#38992,#38993,#38994,#38995,#38996,#38997,#38998,#38999,#39000,#39001,#39002,
#39003,#39004,#39005,#39006),.UNSPECIFIED.,.F.,.F.,(4,1,1,1,1,1,1,1,1,1,
1,1,1,1,1,1,1,4),(6.93617595249389,7.96866100733354,9.0011460621732,10.0336311170129,
10.5498736444327,11.0661161718525,12.0986012266922,13.1310862815318,13.8194096514249,
14.507733021318,15.1960563912111,16.5727031309973,17.2610265008905,17.7772690283103,
18.2935115557301,19.3259966105698,20.3584816654094,21.3909667202491),
 .UNSPECIFIED.);
#218=B_SPLINE_CURVE_WITH_KNOTS('',3,(#39009,#39010,#39011,#39012,#39013,
#39014,#39015,#39016,#39017,#39018,#39019,#39020,#39021,#39022,#39023,#39024,
#39025,#39026,#39027,#39028),.UNSPECIFIED.,.F.,.F.,(4,1,1,1,1,1,1,1,1,1,
1,1,1,1,1,1,1,4),(-21.3909667202491,-20.3584816654094,-19.3259966105698,
-18.2935115557301,-17.7772690283103,-17.2610265008905,-16.5727031309973,
-15.1960563912111,-14.507733021318,-13.8194096514249,-13.1310862815318,
-12.0986012266922,-11.0661161718525,-10.5498736444327,-10.0336311170129,
-9.0011460621732,-7.96866100733354,-6.93617595249389),.UNSPECIFIED.);
#219=B_SPLINE_CURVE_WITH_KNOTS('',3,(#39045,#39046,#39047,#39048),
 .UNSPECIFIED.,.F.,.F.,(4,4),(-6.93617595249389,-6.91671820418794),
 .UNSPECIFIED.);
#220=B_SPLINE_CURVE_WITH_KNOTS('',3,(#39049,#39050,#39051,#39052),
 .UNSPECIFIED.,.F.,.F.,(4,4),(6.91671820418794,6.93617595249389),
 .UNSPECIFIED.);
#221=B_SPLINE_CURVE_WITH_KNOTS('',3,(#39069,#39070,#39071,#39072),
 .UNSPECIFIED.,.F.,.F.,(4,4),(-21.410424468555,-21.3909667202491),
 .UNSPECIFIED.);
#222=B_SPLINE_CURVE_WITH_KNOTS('',3,(#39073,#39074,#39075,#39076),
 .UNSPECIFIED.,.F.,.F.,(4,4),(21.3909667202491,21.410424468555),
 .UNSPECIFIED.);
#223=B_SPLINE_CURVE_WITH_KNOTS('',3,(#39093,#39094,#39095,#39096,#39097,
#39098,#39099),.UNSPECIFIED.,.F.,.F.,(4,3,4),(-0.0722630748993823,-0.0361526280409953,
0.),.UNSPECIFIED.);
#224=B_SPLINE_CURVE_WITH_KNOTS('',3,(#39129,#39130,#39131,#39132,#39133,
#39134,#39135),.UNSPECIFIED.,.F.,.F.,(4,1,1,1,4),(-1.46843716746911,-1.23331881650262,
-0.998200465536129,-0.821861702311259,-0.645522939086389),.UNSPECIFIED.);
#225=B_SPLINE_CURVE_WITH_KNOTS('',3,(#39136,#39137,#39138,#39139,#39140,
#39141,#39142),.UNSPECIFIED.,.F.,.F.,(4,1,1,1,4),(0.651509071335782,0.821861702311259,
0.998200465536129,1.23331881650262,1.46789448307402),.UNSPECIFIED.);
#226=B_SPLINE_CURVE_WITH_KNOTS('',3,(#39147,#39148,#39149,#39150,#39151,
#39152,#39153),.UNSPECIFIED.,.F.,.F.,(4,1,1,1,4),(-1.46789448307312,-1.29209840424425,
-1.11575964101938,-0.880641290052883,-0.651509067467386),.UNSPECIFIED.);
#227=B_SPLINE_CURVE_WITH_KNOTS('',3,(#39158,#39159,#39160,#39161,#39162,
#39163,#39164),.UNSPECIFIED.,.F.,.F.,(4,3,4),(-0.0724895287827058,-0.0362236180763736,
0.),.UNSPECIFIED.);
#228=B_SPLINE_CURVE_WITH_KNOTS('',3,(#39193,#39194,#39195,#39196,#39197,
#39198,#39199),.UNSPECIFIED.,.F.,.F.,(4,1,1,1,4),(0.645522939086389,0.880641290052883,
1.11575964101938,1.29209840424425,1.46843716746912),.UNSPECIFIED.);
#229=B_SPLINE_CURVE_WITH_KNOTS('',3,(#39202,#39203,#39204,#39205,#39206),
 .UNSPECIFIED.,.F.,.F.,(4,1,4),(3.93038111840777,4.35323723299001,4.44759047801891),
 .UNSPECIFIED.);
#230=B_SPLINE_CURVE_WITH_KNOTS('',3,(#39241,#39242,#39243,#39244,#39245,
#39246,#39247,#39248,#39249,#39250,#39251,#39252,#39253,#39254,#39255,#39256,
#39257,#39258,#39259,#39260,#39261,#39262,#39263,#39264,#39265,#39266,#39267,
#39268),.UNSPECIFIED.,.F.,.F.,(4,3,3,3,3,3,3,3,3,4),(-4.91704538576632,
-4.77089990935868,-4.70272379532275,-4.63510958231822,-4.4904291378749,
-4.46686475597115,-4.35321853983198,-4.20436404417231,-4.01903755304543,
-3.93038111840777),.UNSPECIFIED.);
#231=B_SPLINE_CURVE_WITH_KNOTS('',3,(#39301,#39302,#39303,#39304,#39305,
#39306),.UNSPECIFIED.,.F.,.F.,(4,1,1,4),(-1.30436309345028,-0.740554939421754,
-0.599602900914624,-0.317698823900363),.UNSPECIFIED.);
#232=B_SPLINE_CURVE_WITH_KNOTS('',3,(#39307,#39308,#39309,#39310),
 .UNSPECIFIED.,.F.,.F.,(4,4),(0.787258846493104,1.30436309345028),
 .UNSPECIFIED.);
#233=B_SPLINE_CURVE_WITH_KNOTS('',3,(#39348,#39349,#39350,#39351,#39352,
#39353,#39354,#39355,#39356,#39357),.UNSPECIFIED.,.F.,.F.,(4,2,2,2,4),(0.,
0.1527055005571,0.3054110011142,0.458115566811898,0.610820132509595),
 .UNSPECIFIED.);
#234=B_SPLINE_CURVE_WITH_KNOTS('',3,(#39358,#39359,#39360,#39361,#39362,
#39363,#39364,#39365,#39366,#39367,#39368,#39369,#39370,#39371,#39372,#39373,
#39374,#39375,#39376,#39377,#39378,#39379,#39380,#39381,#39382,#39383),
 .UNSPECIFIED.,.F.,.F.,(4,2,2,2,2,2,2,2,2,2,2,2,4),(0.610820132509595,0.763524698207293,
0.916229263904991,1.06893476446209,1.22164026501919,1.37434576557629,1.52705126613339,
1.67975583183109,1.83246039752879,1.98516496322648,2.13786952892418,2.29057502948128,
2.44328053003838),.UNSPECIFIED.);
#235=B_SPLINE_CURVE_WITH_KNOTS('',3,(#39387,#39388,#39389,#39390,#39391,
#39392,#39393,#39394,#39395,#39396,#39397,#39398,#39399,#39400,#39401,#39402,
#39403,#39404,#39405,#39406,#39407,#39408,#39409,#39410,#39411,#39412),
 .UNSPECIFIED.,.F.,.F.,(4,2,2,2,2,2,2,2,2,2,2,2,4),(0.,0.380941401599584,
0.761882803199167,1.14272967212036,1.52357654104155,1.90442340996273,2.28527027888392,
2.66621168048351,3.04715308208309,3.42809448368267,3.80903588528226,4.18988275420345,
4.57072962312464),.UNSPECIFIED.);
#236=B_SPLINE_CURVE_WITH_KNOTS('',3,(#39413,#39414,#39415,#39416,#39417,
#39418,#39419,#39420,#39421,#39422),.UNSPECIFIED.,.F.,.F.,(4,2,2,2,4),(4.57072962312464,
4.95157649204583,5.33242336096701,5.7133647625666,6.09430616416618),
 .UNSPECIFIED.);
#1000=SHAPE_REPRESENTATION_RELATIONSHIP('SRR','None',#76737,#1020);
#1020=ADVANCED_BREP_SHAPE_REPRESENTATION('',(#1060),#76641);
#1040=STYLED_ITEM('',(#76892),#1060);
#1060=MANIFOLD_SOLID_BREP('Casing',#26665);
#1083=TOROIDAL_SURFACE('',#27370,4.8,0.3);
#1084=TOROIDAL_SURFACE('',#27375,5.8,0.3);
#1093=ELLIPSE('',#27339,0.378533806327918,0.3);
#1094=ELLIPSE('',#27353,28.3617829428801,19.3853883884215);
#1095=ELLIPSE('',#27356,28.3617829428803,19.3853883884215);
#1096=ELLIPSE('',#27361,0.378533806327918,0.3);
#1097=ELLIPSE('',#27367,0.424264068711929,0.3);
#1098=ELLIPSE('',#27369,0.424264068711928,0.3);
#1122=CYLINDRICAL_SURFACE('',#27154,1.8);
#1123=CYLINDRICAL_SURFACE('',#27168,0.305);
#1124=CYLINDRICAL_SURFACE('',#27174,0.305);
#1125=CYLINDRICAL_SURFACE('',#27193,5.5);
#1126=CYLINDRICAL_SURFACE('',#27197,0.700000000000003);
#1127=CYLINDRICAL_SURFACE('',#27228,1.);
#1128=CYLINDRICAL_SURFACE('',#27233,0.3);
#1129=CYLINDRICAL_SURFACE('',#27248,0.550000000000001);
#1130=CYLINDRICAL_SURFACE('',#27257,0.550000000000001);
#1131=CYLINDRICAL_SURFACE('',#27266,0.550000000000001);
#1132=CYLINDRICAL_SURFACE('',#27275,0.550000000000001);
#1133=CYLINDRICAL_SURFACE('',#27283,0.305);
#1134=CYLINDRICAL_SURFACE('',#27289,0.305);
#1135=CYLINDRICAL_SURFACE('',#27298,0.550000000000001);
#1136=CYLINDRICAL_SURFACE('',#27315,0.550000000000001);
#1137=CYLINDRICAL_SURFACE('',#27321,0.550000000000001);
#1138=CYLINDRICAL_SURFACE('',#27327,0.550000000000001);
#1139=CYLINDRICAL_SURFACE('',#27338,0.3);
#1140=CYLINDRICAL_SURFACE('',#27340,1.);
#1141=CYLINDRICAL_SURFACE('',#27342,1.);
#1142=CYLINDRICAL_SURFACE('',#27349,4.5);
#1143=CYLINDRICAL_SURFACE('',#27355,19.3853883884215);
#1144=CYLINDRICAL_SURFACE('',#27359,0.3);
#1145=CYLINDRICAL_SURFACE('',#27363,0.3);
#1146=CYLINDRICAL_SURFACE('',#27365,0.3);
#1147=CYLINDRICAL_SURFACE('',#27368,0.3);
#1148=CYLINDRICAL_SURFACE('',#27372,0.3);
#1149=CYLINDRICAL_SURFACE('',#27373,0.3);
#1150=CYLINDRICAL_SURFACE('',#27374,1.);
#1151=CYLINDRICAL_SURFACE('',#27386,0.405000000000001);
#1152=CYLINDRICAL_SURFACE('',#27387,1.005);
#1153=CYLINDRICAL_SURFACE('',#27391,0.605000000000004);
#1154=CYLINDRICAL_SURFACE('',#27392,3.5);
#1561=FACE_BOUND('',#4233,.T.);
#1562=FACE_BOUND('',#4243,.T.);
#1563=FACE_BOUND('',#4244,.T.);
#1564=FACE_BOUND('',#4250,.T.);
#1565=FACE_BOUND('',#4253,.T.);
#1566=FACE_BOUND('',#4254,.T.);
#1567=FACE_BOUND('',#4255,.T.);
#1568=FACE_BOUND('',#4286,.T.);
#1569=FACE_BOUND('',#4292,.T.);
#1570=FACE_BOUND('',#4293,.T.);
#1571=FACE_BOUND('',#4328,.T.);
#1572=FACE_BOUND('',#4329,.T.);
#1573=FACE_BOUND('',#4330,.T.);
#1574=FACE_BOUND('',#4331,.T.);
#1575=FACE_BOUND('',#4401,.T.);
#1576=FACE_BOUND('',#4405,.T.);
#1577=FACE_BOUND('',#4408,.T.);
#1578=FACE_BOUND('',#4409,.T.);
#1579=FACE_BOUND('',#4411,.T.);
#1737=PLANE('',#27149);
#1738=PLANE('',#27176);
#1739=PLANE('',#27177);
#1740=PLANE('',#27184);
#1741=PLANE('',#27185);
#1742=PLANE('',#27191);
#1743=PLANE('',#27200);
#1744=PLANE('',#27201);
#1745=PLANE('',#27205);
#1746=PLANE('',#27206);
#1747=PLANE('',#27207);
#1748=PLANE('',#27208);
#1749=PLANE('',#27209);
#1750=PLANE('',#27210);
#1751=PLANE('',#27214);
#1752=PLANE('',#27218);
#1753=PLANE('',#27219);
#1754=PLANE('',#27220);
#1755=PLANE('',#27221);
#1756=PLANE('',#27222);
#1757=PLANE('',#27227);
#1758=PLANE('',#27230);
#1759=PLANE('',#27234);
#1760=PLANE('',#27235);
#1761=PLANE('',#27236);
#1762=PLANE('',#27237);
#1763=PLANE('',#27242);
#1764=PLANE('',#27245);
#1765=PLANE('',#27250);
#1766=PLANE('',#27251);
#1767=PLANE('',#27254);
#1768=PLANE('',#27259);
#1769=PLANE('',#27260);
#1770=PLANE('',#27263);
#1771=PLANE('',#27268);
#1772=PLANE('',#27269);
#1773=PLANE('',#27272);
#1774=PLANE('',#27277);
#1775=PLANE('',#27291);
#1776=PLANE('',#27295);
#1777=PLANE('',#27299);
#1778=PLANE('',#27310);
#1779=PLANE('',#27313);
#1780=PLANE('',#27316);
#1781=PLANE('',#27319);
#1782=PLANE('',#27322);
#1783=PLANE('',#27325);
#1784=PLANE('',#27330);
#1785=PLANE('',#27333);
#1786=PLANE('',#27336);
#1787=PLANE('',#27341);
#1788=PLANE('',#27343);
#1789=PLANE('',#27344);
#1790=PLANE('',#27348);
#1791=PLANE('',#27351);
#1792=PLANE('',#27352);
#1793=PLANE('',#27354);
#1794=PLANE('',#27357);
#1795=PLANE('',#27358);
#1796=PLANE('',#27364);
#1797=PLANE('',#27376);
#1798=PLANE('',#27377);
#1799=PLANE('',#27378);
#1800=PLANE('',#27379);
#1801=PLANE('',#27384);
#1802=PLANE('',#27389);
#1803=PLANE('',#27394);
#2670=FACE_OUTER_BOUND('',#4230,.T.);
#2671=FACE_OUTER_BOUND('',#4231,.T.);
#2672=FACE_OUTER_BOUND('',#4232,.T.);
#2673=FACE_OUTER_BOUND('',#4234,.T.);
#2674=FACE_OUTER_BOUND('',#4235,.T.);
#2675=FACE_OUTER_BOUND('',#4236,.T.);
#2676=FACE_OUTER_BOUND('',#4237,.T.);
#2677=FACE_OUTER_BOUND('',#4238,.T.);
#2678=FACE_OUTER_BOUND('',#4239,.T.);
#2679=FACE_OUTER_BOUND('',#4240,.T.);
#2680=FACE_OUTER_BOUND('',#4241,.T.);
#2681=FACE_OUTER_BOUND('',#4242,.T.);
#2682=FACE_OUTER_BOUND('',#4245,.T.);
#2683=FACE_OUTER_BOUND('',#4246,.T.);
#2684=FACE_OUTER_BOUND('',#4247,.T.);
#2685=FACE_OUTER_BOUND('',#4248,.T.);
#2686=FACE_OUTER_BOUND('',#4249,.T.);
#2687=FACE_OUTER_BOUND('',#4251,.T.);
#2688=FACE_OUTER_BOUND('',#4252,.T.);
#2689=FACE_OUTER_BOUND('',#4256,.T.);
#2690=FACE_OUTER_BOUND('',#4257,.T.);
#2691=FACE_OUTER_BOUND('',#4258,.T.);
#2692=FACE_OUTER_BOUND('',#4259,.T.);
#2693=FACE_OUTER_BOUND('',#4260,.T.);
#2694=FACE_OUTER_BOUND('',#4261,.T.);
#2695=FACE_OUTER_BOUND('',#4262,.T.);
#2696=FACE_OUTER_BOUND('',#4263,.T.);
#2697=FACE_OUTER_BOUND('',#4264,.T.);
#2698=FACE_OUTER_BOUND('',#4265,.T.);
#2699=FACE_OUTER_BOUND('',#4266,.T.);
#2700=FACE_OUTER_BOUND('',#4267,.T.);
#2701=FACE_OUTER_BOUND('',#4268,.T.);
#2702=FACE_OUTER_BOUND('',#4269,.T.);
#2703=FACE_OUTER_BOUND('',#4270,.T.);
#2704=FACE_OUTER_BOUND('',#4271,.T.);
#2705=FACE_OUTER_BOUND('',#4272,.T.);
#2706=FACE_OUTER_BOUND('',#4273,.T.);
#2707=FACE_OUTER_BOUND('',#4274,.T.);
#2708=FACE_OUTER_BOUND('',#4275,.T.);
#2709=FACE_OUTER_BOUND('',#4276,.T.);
#2710=FACE_OUTER_BOUND('',#4277,.T.);
#2711=FACE_OUTER_BOUND('',#4278,.T.);
#2712=FACE_OUTER_BOUND('',#4279,.T.);
#2713=FACE_OUTER_BOUND('',#4280,.T.);
#2714=FACE_OUTER_BOUND('',#4281,.T.);
#2715=FACE_OUTER_BOUND('',#4282,.T.);
#2716=FACE_OUTER_BOUND('',#4283,.T.);
#2717=FACE_OUTER_BOUND('',#4284,.T.);
#2718=FACE_OUTER_BOUND('',#4285,.T.);
#2719=FACE_OUTER_BOUND('',#4287,.T.);
#2720=FACE_OUTER_BOUND('',#4288,.T.);
#2721=FACE_OUTER_BOUND('',#4289,.T.);
#2722=FACE_OUTER_BOUND('',#4290,.T.);
#2723=FACE_OUTER_BOUND('',#4291,.T.);
#2724=FACE_OUTER_BOUND('',#4294,.T.);
#2725=FACE_OUTER_BOUND('',#4295,.T.);
#2726=FACE_OUTER_BOUND('',#4296,.T.);
#2727=FACE_OUTER_BOUND('',#4297,.T.);
#2728=FACE_OUTER_BOUND('',#4298,.T.);
#2729=FACE_OUTER_BOUND('',#4299,.T.);
#2730=FACE_OUTER_BOUND('',#4300,.T.);
#2731=FACE_OUTER_BOUND('',#4301,.T.);
#2732=FACE_OUTER_BOUND('',#4302,.T.);
#2733=FACE_OUTER_BOUND('',#4303,.T.);
#2734=FACE_OUTER_BOUND('',#4304,.T.);
#2735=FACE_OUTER_BOUND('',#4305,.T.);
#2736=FACE_OUTER_BOUND('',#4306,.T.);
#2737=FACE_OUTER_BOUND('',#4307,.T.);
#2738=FACE_OUTER_BOUND('',#4308,.T.);
#2739=FACE_OUTER_BOUND('',#4309,.T.);
#2740=FACE_OUTER_BOUND('',#4310,.T.);
#2741=FACE_OUTER_BOUND('',#4311,.T.);
#2742=FACE_OUTER_BOUND('',#4312,.T.);
#2743=FACE_OUTER_BOUND('',#4313,.T.);
#2744=FACE_OUTER_BOUND('',#4314,.T.);
#2745=FACE_OUTER_BOUND('',#4315,.T.);
#2746=FACE_OUTER_BOUND('',#4316,.T.);
#2747=FACE_OUTER_BOUND('',#4317,.T.);
#2748=FACE_OUTER_BOUND('',#4318,.T.);
#2749=FACE_OUTER_BOUND('',#4319,.T.);
#2750=FACE_OUTER_BOUND('',#4320,.T.);
#2751=FACE_OUTER_BOUND('',#4321,.T.);
#2752=FACE_OUTER_BOUND('',#4322,.T.);
#2753=FACE_OUTER_BOUND('',#4323,.T.);
#2754=FACE_OUTER_BOUND('',#4324,.T.);
#2755=FACE_OUTER_BOUND('',#4325,.T.);
#2756=FACE_OUTER_BOUND('',#4326,.T.);
#2757=FACE_OUTER_BOUND('',#4327,.T.);
#2758=FACE_OUTER_BOUND('',#4332,.T.);
#2759=FACE_OUTER_BOUND('',#4333,.T.);
#2760=FACE_OUTER_BOUND('',#4334,.T.);
#2761=FACE_OUTER_BOUND('',#4335,.T.);
#2762=FACE_OUTER_BOUND('',#4336,.T.);
#2763=FACE_OUTER_BOUND('',#4337,.T.);
#2764=FACE_OUTER_BOUND('',#4338,.T.);
#2765=FACE_OUTER_BOUND('',#4339,.T.);
#2766=FACE_OUTER_BOUND('',#4340,.T.);
#2767=FACE_OUTER_BOUND('',#4341,.T.);
#2768=FACE_OUTER_BOUND('',#4342,.T.);
#2769=FACE_OUTER_BOUND('',#4343,.T.);
#2770=FACE_OUTER_BOUND('',#4344,.T.);
#2771=FACE_OUTER_BOUND('',#4345,.T.);
#2772=FACE_OUTER_BOUND('',#4346,.T.);
#2773=FACE_OUTER_BOUND('',#4347,.T.);
#2774=FACE_OUTER_BOUND('',#4348,.T.);
#2775=FACE_OUTER_BOUND('',#4349,.T.);
#2776=FACE_OUTER_BOUND('',#4350,.T.);
#2777=FACE_OUTER_BOUND('',#4351,.T.);
#2778=FACE_OUTER_BOUND('',#4352,.T.);
#2779=FACE_OUTER_BOUND('',#4353,.T.);
#2780=FACE_OUTER_BOUND('',#4354,.T.);
#2781=FACE_OUTER_BOUND('',#4355,.T.);
#2782=FACE_OUTER_BOUND('',#4356,.T.);
#2783=FACE_OUTER_BOUND('',#4357,.T.);
#2784=FACE_OUTER_BOUND('',#4358,.T.);
#2785=FACE_OUTER_BOUND('',#4359,.T.);
#2786=FACE_OUTER_BOUND('',#4360,.T.);
#2787=FACE_OUTER_BOUND('',#4361,.T.);
#2788=FACE_OUTER_BOUND('',#4362,.T.);
#2789=FACE_OUTER_BOUND('',#4363,.T.);
#2790=FACE_OUTER_BOUND('',#4364,.T.);
#2791=FACE_OUTER_BOUND('',#4365,.T.);
#2792=FACE_OUTER_BOUND('',#4366,.T.);
#2793=FACE_OUTER_BOUND('',#4367,.T.);
#2794=FACE_OUTER_BOUND('',#4368,.T.);
#2795=FACE_OUTER_BOUND('',#4369,.T.);
#2796=FACE_OUTER_BOUND('',#4370,.T.);
#2797=FACE_OUTER_BOUND('',#4371,.T.);
#2798=FACE_OUTER_BOUND('',#4372,.T.);
#2799=FACE_OUTER_BOUND('',#4373,.T.);
#2800=FACE_OUTER_BOUND('',#4374,.T.);
#2801=FACE_OUTER_BOUND('',#4375,.T.);
#2802=FACE_OUTER_BOUND('',#4376,.T.);
#2803=FACE_OUTER_BOUND('',#4377,.T.);
#2804=FACE_OUTER_BOUND('',#4378,.T.);
#2805=FACE_OUTER_BOUND('',#4379,.T.);
#2806=FACE_OUTER_BOUND('',#4380,.T.);
#2807=FACE_OUTER_BOUND('',#4381,.T.);
#2808=FACE_OUTER_BOUND('',#4382,.T.);
#2809=FACE_OUTER_BOUND('',#4383,.T.);
#2810=FACE_OUTER_BOUND('',#4384,.T.);
#2811=FACE_OUTER_BOUND('',#4385,.T.);
#2812=FACE_OUTER_BOUND('',#4386,.T.);
#2813=FACE_OUTER_BOUND('',#4387,.T.);
#2814=FACE_OUTER_BOUND('',#4388,.T.);
#2815=FACE_OUTER_BOUND('',#4389,.T.);
#2816=FACE_OUTER_BOUND('',#4390,.T.);
#2817=FACE_OUTER_BOUND('',#4391,.T.);
#2818=FACE_OUTER_BOUND('',#4392,.T.);
#2819=FACE_OUTER_BOUND('',#4393,.T.);
#2820=FACE_OUTER_BOUND('',#4394,.T.);
#2821=FACE_OUTER_BOUND('',#4395,.T.);
#2822=FACE_OUTER_BOUND('',#4396,.T.);
#2823=FACE_OUTER_BOUND('',#4397,.T.);
#2824=FACE_OUTER_BOUND('',#4398,.T.);
#2825=FACE_OUTER_BOUND('',#4399,.T.);
#2826=FACE_OUTER_BOUND('',#4400,.T.);
#2827=FACE_OUTER_BOUND('',#4402,.T.);
#2828=FACE_OUTER_BOUND('',#4403,.T.);
#2829=FACE_OUTER_BOUND('',#4404,.T.);
#2830=FACE_OUTER_BOUND('',#4406,.T.);
#2831=FACE_OUTER_BOUND('',#4407,.T.);
#2832=FACE_OUTER_BOUND('',#4410,.T.);
#4230=EDGE_LOOP('',(#17837,#17838,#17839,#17840,#17841));
#4231=EDGE_LOOP('',(#17842,#17843,#17844,#17845,#17846,#17847));
#4232=EDGE_LOOP('',(#17848));
#4233=EDGE_LOOP('',(#17849));
#4234=EDGE_LOOP('',(#17850,#17851,#17852,#17853,#17854,#17855));
#4235=EDGE_LOOP('',(#17856,#17857,#17858,#17859,#17860,#17861));
#4236=EDGE_LOOP('',(#17862,#17863,#17864,#17865,#17866,#17867,#17868));
#4237=EDGE_LOOP('',(#17869,#17870,#17871,#17872,#17873,#17874,#17875,#17876,
#17877,#17878,#17879,#17880,#17881));
#4238=EDGE_LOOP('',(#17882,#17883,#17884,#17885,#17886));
#4239=EDGE_LOOP('',(#17887,#17888,#17889,#17890,#17891,#17892));
#4240=EDGE_LOOP('',(#17893,#17894,#17895,#17896));
#4241=EDGE_LOOP('',(#17897,#17898,#17899,#17900,#17901,#17902));
#4242=EDGE_LOOP('',(#17903,#17904,#17905,#17906,#17907,#17908,#17909,#17910));
#4243=EDGE_LOOP('',(#17911,#17912,#17913,#17914));
#4244=EDGE_LOOP('',(#17915,#17916,#17917,#17918));
#4245=EDGE_LOOP('',(#17919,#17920,#17921,#17922,#17923));
#4246=EDGE_LOOP('',(#17924,#17925,#17926,#17927,#17928));
#4247=EDGE_LOOP('',(#17929,#17930,#17931,#17932));
#4248=EDGE_LOOP('',(#17933,#17934,#17935,#17936));
#4249=EDGE_LOOP('',(#17937));
#4250=EDGE_LOOP('',(#17938));
#4251=EDGE_LOOP('',(#17939,#17940,#17941,#17942,#17943));
#4252=EDGE_LOOP('',(#17944,#17945,#17946,#17947,#17948,#17949));
#4253=EDGE_LOOP('',(#17950,#17951,#17952,#17953,#17954,#17955,#17956,#17957));
#4254=EDGE_LOOP('',(#17958,#17959));
#4255=EDGE_LOOP('',(#17960));
#4256=EDGE_LOOP('',(#17961,#17962,#17963,#17964,#17965));
#4257=EDGE_LOOP('',(#17966,#17967,#17968,#17969,#17970));
#4258=EDGE_LOOP('',(#17971,#17972,#17973,#17974));
#4259=EDGE_LOOP('',(#17975,#17976,#17977,#17978));
#4260=EDGE_LOOP('',(#17979,#17980,#17981,#17982));
#4261=EDGE_LOOP('',(#17983,#17984,#17985,#17986));
#4262=EDGE_LOOP('',(#17987,#17988,#17989,#17990));
#4263=EDGE_LOOP('',(#17991,#17992,#17993,#17994));
#4264=EDGE_LOOP('',(#17995,#17996,#17997,#17998,#17999));
#4265=EDGE_LOOP('',(#18000,#18001,#18002,#18003,#18004));
#4266=EDGE_LOOP('',(#18005,#18006,#18007));
#4267=EDGE_LOOP('',(#18008,#18009,#18010,#18011));
#4268=EDGE_LOOP('',(#18012,#18013,#18014));
#4269=EDGE_LOOP('',(#18015,#18016,#18017,#18018));
#4270=EDGE_LOOP('',(#18019,#18020,#18021,#18022));
#4271=EDGE_LOOP('',(#18023,#18024,#18025,#18026));
#4272=EDGE_LOOP('',(#18027,#18028,#18029,#18030));
#4273=EDGE_LOOP('',(#18031,#18032,#18033,#18034));
#4274=EDGE_LOOP('',(#18035,#18036,#18037,#18038));
#4275=EDGE_LOOP('',(#18039,#18040,#18041,#18042));
#4276=EDGE_LOOP('',(#18043,#18044,#18045,#18046));
#4277=EDGE_LOOP('',(#18047,#18048,#18049,#18050));
#4278=EDGE_LOOP('',(#18051,#18052,#18053,#18054));
#4279=EDGE_LOOP('',(#18055,#18056,#18057,#18058));
#4280=EDGE_LOOP('',(#18059,#18060,#18061,#18062));
#4281=EDGE_LOOP('',(#18063,#18064,#18065,#18066));
#4282=EDGE_LOOP('',(#18067,#18068,#18069,#18070));
#4283=EDGE_LOOP('',(#18071,#18072,#18073,#18074,#18075,#18076,#18077,#18078));
#4284=EDGE_LOOP('',(#18079,#18080,#18081,#18082,#18083,#18084,#18085,#18086,
#18087,#18088));
#4285=EDGE_LOOP('',(#18089,#18090,#18091,#18092,#18093,#18094,#18095,#18096,
#18097,#18098,#18099,#18100));
#4286=EDGE_LOOP('',(#18101,#18102,#18103,#18104));
#4287=EDGE_LOOP('',(#18105,#18106,#18107,#18108,#18109,#18110));
#4288=EDGE_LOOP('',(#18111,#18112,#18113,#18114));
#4289=EDGE_LOOP('',(#18115,#18116,#18117,#18118));
#4290=EDGE_LOOP('',(#18119,#18120,#18121,#18122));
#4291=EDGE_LOOP('',(#18123,#18124,#18125,#18126,#18127,#18128));
#4292=EDGE_LOOP('',(#18129,#18130,#18131,#18132));
#4293=EDGE_LOOP('',(#18133,#18134,#18135,#18136));
#4294=EDGE_LOOP('',(#18137,#18138,#18139,#18140));
#4295=EDGE_LOOP('',(#18141,#18142,#18143,#18144));
#4296=EDGE_LOOP('',(#18145,#18146,#18147,#18148));
#4297=EDGE_LOOP('',(#18149,#18150,#18151,#18152));
#4298=EDGE_LOOP('',(#18153,#18154,#18155,#18156));
#4299=EDGE_LOOP('',(#18157,#18158,#18159,#18160));
#4300=EDGE_LOOP('',(#18161,#18162,#18163,#18164));
#4301=EDGE_LOOP('',(#18165,#18166,#18167,#18168));
#4302=EDGE_LOOP('',(#18169,#18170,#18171,#18172));
#4303=EDGE_LOOP('',(#18173,#18174,#18175,#18176));
#4304=EDGE_LOOP('',(#18177,#18178,#18179,#18180));
#4305=EDGE_LOOP('',(#18181,#18182,#18183,#18184));
#4306=EDGE_LOOP('',(#18185,#18186,#18187,#18188));
#4307=EDGE_LOOP('',(#18189,#18190,#18191,#18192));
#4308=EDGE_LOOP('',(#18193,#18194,#18195,#18196));
#4309=EDGE_LOOP('',(#18197,#18198,#18199,#18200));
#4310=EDGE_LOOP('',(#18201,#18202,#18203,#18204));
#4311=EDGE_LOOP('',(#18205,#18206,#18207,#18208));
#4312=EDGE_LOOP('',(#18209,#18210,#18211,#18212));
#4313=EDGE_LOOP('',(#18213,#18214,#18215,#18216));
#4314=EDGE_LOOP('',(#18217,#18218,#18219,#18220));
#4315=EDGE_LOOP('',(#18221,#18222,#18223,#18224));
#4316=EDGE_LOOP('',(#18225,#18226,#18227,#18228));
#4317=EDGE_LOOP('',(#18229,#18230,#18231,#18232));
#4318=EDGE_LOOP('',(#18233,#18234,#18235,#18236,#18237,#18238,#18239));
#4319=EDGE_LOOP('',(#18240,#18241,#18242,#18243,#18244));
#4320=EDGE_LOOP('',(#18245,#18246,#18247,#18248,#18249,#18250));
#4321=EDGE_LOOP('',(#18251,#18252,#18253,#18254));
#4322=EDGE_LOOP('',(#18255,#18256,#18257,#18258));
#4323=EDGE_LOOP('',(#18259,#18260,#18261,#18262));
#4324=EDGE_LOOP('',(#18263,#18264,#18265,#18266));
#4325=EDGE_LOOP('',(#18267,#18268,#18269,#18270));
#4326=EDGE_LOOP('',(#18271,#18272,#18273,#18274));
#4327=EDGE_LOOP('',(#18275,#18276,#18277,#18278,#18279,#18280,#18281,#18282,
#18283,#18284,#18285,#18286,#18287,#18288,#18289,#18290,#18291,#18292,#18293,
#18294,#18295,#18296));
#4328=EDGE_LOOP('',(#18297,#18298,#18299,#18300));
#4329=EDGE_LOOP('',(#18301,#18302,#18303,#18304));
#4330=EDGE_LOOP('',(#18305,#18306,#18307,#18308));
#4331=EDGE_LOOP('',(#18309,#18310,#18311,#18312));
#4332=EDGE_LOOP('',(#18313,#18314,#18315,#18316));
#4333=EDGE_LOOP('',(#18317,#18318,#18319,#18320));
#4334=EDGE_LOOP('',(#18321,#18322,#18323,#18324));
#4335=EDGE_LOOP('',(#18325,#18326,#18327,#18328));
#4336=EDGE_LOOP('',(#18329,#18330,#18331,#18332));
#4337=EDGE_LOOP('',(#18333,#18334,#18335,#18336));
#4338=EDGE_LOOP('',(#18337,#18338,#18339,#18340));
#4339=EDGE_LOOP('',(#18341,#18342,#18343,#18344));
#4340=EDGE_LOOP('',(#18345,#18346,#18347,#18348));
#4341=EDGE_LOOP('',(#18349,#18350,#18351,#18352));
#4342=EDGE_LOOP('',(#18353,#18354,#18355,#18356));
#4343=EDGE_LOOP('',(#18357,#18358,#18359,#18360));
#4344=EDGE_LOOP('',(#18361,#18362,#18363,#18364));
#4345=EDGE_LOOP('',(#18365,#18366,#18367,#18368));
#4346=EDGE_LOOP('',(#18369,#18370,#18371,#18372));
#4347=EDGE_LOOP('',(#18373,#18374,#18375,#18376));
#4348=EDGE_LOOP('',(#18377,#18378,#18379,#18380));
#4349=EDGE_LOOP('',(#18381,#18382,#18383,#18384));
#4350=EDGE_LOOP('',(#18385,#18386,#18387,#18388));
#4351=EDGE_LOOP('',(#18389,#18390,#18391,#18392));
#4352=EDGE_LOOP('',(#18393,#18394,#18395,#18396));
#4353=EDGE_LOOP('',(#18397,#18398,#18399,#18400));
#4354=EDGE_LOOP('',(#18401,#18402,#18403,#18404));
#4355=EDGE_LOOP('',(#18405,#18406,#18407,#18408));
#4356=EDGE_LOOP('',(#18409,#18410,#18411,#18412));
#4357=EDGE_LOOP('',(#18413,#18414,#18415,#18416));
#4358=EDGE_LOOP('',(#18417,#18418,#18419,#18420));
#4359=EDGE_LOOP('',(#18421,#18422,#18423,#18424));
#4360=EDGE_LOOP('',(#18425,#18426,#18427,#18428,#18429));
#4361=EDGE_LOOP('',(#18430,#18431,#18432,#18433));
#4362=EDGE_LOOP('',(#18434,#18435,#18436,#18437));
#4363=EDGE_LOOP('',(#18438,#18439,#18440,#18441));
#4364=EDGE_LOOP('',(#18442,#18443,#18444,#18445,#18446,#18447,#18448,#18449));
#4365=EDGE_LOOP('',(#18450,#18451,#18452,#18453));
#4366=EDGE_LOOP('',(#18454,#18455,#18456,#18457));
#4367=EDGE_LOOP('',(#18458,#18459,#18460,#18461));
#4368=EDGE_LOOP('',(#18462,#18463,#18464,#18465));
#4369=EDGE_LOOP('',(#18466,#18467,#18468,#18469));
#4370=EDGE_LOOP('',(#18470,#18471,#18472,#18473,#18474,#18475));
#4371=EDGE_LOOP('',(#18476,#18477,#18478,#18479));
#4372=EDGE_LOOP('',(#18480,#18481,#18482,#18483,#18484,#18485));
#4373=EDGE_LOOP('',(#18486,#18487,#18488,#18489,#18490));
#4374=EDGE_LOOP('',(#18491,#18492,#18493,#18494));
#4375=EDGE_LOOP('',(#18495,#18496,#18497,#18498));
#4376=EDGE_LOOP('',(#18499,#18500,#18501,#18502,#18503,#18504,#18505,#18506,
#18507,#18508,#18509,#18510));
#4377=EDGE_LOOP('',(#18511,#18512,#18513,#18514,#18515));
#4378=EDGE_LOOP('',(#18516,#18517,#18518,#18519));
#4379=EDGE_LOOP('',(#18520,#18521,#18522,#18523,#18524,#18525));
#4380=EDGE_LOOP('',(#18526,#18527,#18528,#18529));
#4381=EDGE_LOOP('',(#18530,#18531,#18532,#18533));
#4382=EDGE_LOOP('',(#18534,#18535,#18536,#18537));
#4383=EDGE_LOOP('',(#18538,#18539,#18540,#18541));
#4384=EDGE_LOOP('',(#18542,#18543,#18544,#18545,#18546,#18547));
#4385=EDGE_LOOP('',(#18548,#18549,#18550,#18551));
#4386=EDGE_LOOP('',(#18552,#18553,#18554,#18555));
#4387=EDGE_LOOP('',(#18556,#18557,#18558,#18559));
#4388=EDGE_LOOP('',(#18560,#18561,#18562,#18563));
#4389=EDGE_LOOP('',(#18564,#18565,#18566,#18567,#18568));
#4390=EDGE_LOOP('',(#18569,#18570,#18571,#18572,#18573,#18574,#18575,#18576,
#18577,#18578));
#4391=EDGE_LOOP('',(#18579,#18580,#18581,#18582));
#4392=EDGE_LOOP('',(#18583,#18584,#18585,#18586));
#4393=EDGE_LOOP('',(#18587,#18588,#18589,#18590));
#4394=EDGE_LOOP('',(#18591,#18592,#18593,#18594));
#4395=EDGE_LOOP('',(#18595,#18596,#18597,#18598));
#4396=EDGE_LOOP('',(#18599,#18600,#18601));
#4397=EDGE_LOOP('',(#18602,#18603,#18604));
#4398=EDGE_LOOP('',(#18605,#18606,#18607));
#4399=EDGE_LOOP('',(#18608,#18609,#18610));
#4400=EDGE_LOOP('',(#18611));
#4401=EDGE_LOOP('',(#18612));
#4402=EDGE_LOOP('',(#18613,#18614,#18615,#18616,#18617));
#4403=EDGE_LOOP('',(#18618,#18619,#18620,#18621,#18622));
#4404=EDGE_LOOP('',(#18623));
#4405=EDGE_LOOP('',(#18624));
#4406=EDGE_LOOP('',(#18625,#18626,#18627,#18628));
#4407=EDGE_LOOP('',(#18629,#18630,#18631,#18632));
#4408=EDGE_LOOP('',(#18633,#18634));
#4409=EDGE_LOOP('',(#18635,#18636));
#4410=EDGE_LOOP('',(#18637,#18638,#18639,#18640,#18641,#18642,#18643,#18644,
#18645,#18646,#18647,#18648,#18649));
#4411=EDGE_LOOP('',(#18650));
#5815=CIRCLE('',#27143,1.65000000000001);
#5816=CIRCLE('',#27144,1.73535533905934);
#5817=CIRCLE('',#27145,1.73535533905934);
#5818=CIRCLE('',#27147,1.76464466094067);
#5819=CIRCLE('',#27148,1.76464466094067);
#5820=CIRCLE('',#27150,0.605000000000004);
#5821=CIRCLE('',#27152,1.8);
#5822=CIRCLE('',#27153,1.8);
#5823=CIRCLE('',#27156,0.355000000000002);
#5824=CIRCLE('',#27157,0.305);
#5825=CIRCLE('',#27158,0.305);
#5826=CIRCLE('',#27159,0.355000000000002);
#5827=CIRCLE('',#27161,5.5);
#5828=CIRCLE('',#27162,5.5);
#5829=CIRCLE('',#27163,5.3);
#5830=CIRCLE('',#27164,5.3);
#5831=CIRCLE('',#27165,5.3);
#5832=CIRCLE('',#27166,5.3);
#5833=CIRCLE('',#27167,5.3);
#5834=CIRCLE('',#27169,0.305);
#5835=CIRCLE('',#27171,0.354999999999998);
#5836=CIRCLE('',#27172,0.305);
#5837=CIRCLE('',#27173,0.354999999999998);
#5838=CIRCLE('',#27175,0.305);
#5839=CIRCLE('',#27178,0.95);
#5840=CIRCLE('',#27179,0.950000000000001);
#5841=CIRCLE('',#27180,0.600000000000001);
#5842=CIRCLE('',#27181,0.600000000000001);
#5843=CIRCLE('',#27182,0.600000000000001);
#5844=CIRCLE('',#27183,0.600000000000001);
#5845=CIRCLE('',#27187,5.33535533905933);
#5846=CIRCLE('',#27188,5.25);
#5847=CIRCLE('',#27190,5.46464466094067);
#5848=CIRCLE('',#27192,3.5);
#5849=CIRCLE('',#27194,5.5);
#5850=CIRCLE('',#27195,5.5);
#5851=CIRCLE('',#27196,5.5);
#5852=CIRCLE('',#27198,0.700000000000003);
#5853=CIRCLE('',#27203,19.3353883884215);
#5854=CIRCLE('',#27204,19.3853883884215);
#5855=CIRCLE('',#27212,1.);
#5856=CIRCLE('',#27213,0.95);
#5857=CIRCLE('',#27216,1.);
#5858=CIRCLE('',#27217,0.95);
#5859=CIRCLE('',#27224,1.);
#5860=CIRCLE('',#27226,1.);
#5861=CIRCLE('',#27229,1.);
#5862=CIRCLE('',#27231,5.8);
#5863=CIRCLE('',#27232,4.8);
#5864=CIRCLE('',#27238,0.600000000000001);
#5865=CIRCLE('',#27239,0.600000000000001);
#5866=CIRCLE('',#27240,0.600000000000001);
#5867=CIRCLE('',#27241,0.600000000000001);
#5868=CIRCLE('',#27244,0.550000000000001);
#5869=CIRCLE('',#27247,0.550000000000001);
#5870=CIRCLE('',#27249,0.550000000000001);
#5871=CIRCLE('',#27253,0.550000000000001);
#5872=CIRCLE('',#27256,0.550000000000001);
#5873=CIRCLE('',#27258,0.550000000000001);
#5874=CIRCLE('',#27262,0.550000000000001);
#5875=CIRCLE('',#27265,0.550000000000001);
#5876=CIRCLE('',#27267,0.550000000000001);
#5877=CIRCLE('',#27271,0.550000000000001);
#5878=CIRCLE('',#27274,0.550000000000001);
#5879=CIRCLE('',#27276,0.550000000000001);
#5880=CIRCLE('',#27279,0.355000000000002);
#5881=CIRCLE('',#27280,0.305);
#5882=CIRCLE('',#27281,0.305);
#5883=CIRCLE('',#27282,0.355000000000002);
#5884=CIRCLE('',#27284,0.305);
#5885=CIRCLE('',#27286,0.355000000000001);
#5886=CIRCLE('',#27287,0.305);
#5887=CIRCLE('',#27288,0.355000000000001);
#5888=CIRCLE('',#27290,0.305);
#5889=CIRCLE('',#27293,0.600000000000001);
#5890=CIRCLE('',#27294,0.550000000000001);
#5891=CIRCLE('',#27297,0.600000000000001);
#5892=CIRCLE('',#27300,0.95);
#5893=CIRCLE('',#27301,0.95);
#5894=CIRCLE('',#27302,0.95);
#5895=CIRCLE('',#27303,0.950000000000001);
#5896=CIRCLE('',#27304,0.600000000000001);
#5897=CIRCLE('',#27305,0.600000000000001);
#5898=CIRCLE('',#27306,0.600000000000001);
#5899=CIRCLE('',#27307,0.600000000000001);
#5900=CIRCLE('',#27308,0.600000000000001);
#5901=CIRCLE('',#27309,0.600000000000001);
#5902=CIRCLE('',#27312,0.550000000000001);
#5903=CIRCLE('',#27318,0.550000000000001);
#5904=CIRCLE('',#27324,0.550000000000001);
#5905=CIRCLE('',#27329,1.);
#5906=CIRCLE('',#27332,1.);
#5907=CIRCLE('',#27335,1.);
#5908=CIRCLE('',#27346,19.3853883884215);
#5909=CIRCLE('',#27347,19.3353883884215);
#5910=CIRCLE('',#27350,4.5);
#5911=CIRCLE('',#27360,0.299999999999999);
#5912=CIRCLE('',#27362,0.3);
#5913=CIRCLE('',#27366,0.3);
#5914=CIRCLE('',#27371,0.3);
#5915=CIRCLE('',#27385,0.405000000000001);
#5916=CIRCLE('',#27388,1.005);
#5917=CIRCLE('',#27390,0.605000000000004);
#5918=CIRCLE('',#27393,3.5);
#6830=LINE('',#37044,#8986);
#6831=LINE('',#37050,#8987);
#6832=LINE('',#37059,#8988);
#6833=LINE('',#37065,#8989);
#6834=LINE('',#37147,#8990);
#6835=LINE('',#37158,#8991);
#6836=LINE('',#37191,#8992);
#6837=LINE('',#37196,#8993);
#6838=LINE('',#37202,#8994);
#6839=LINE('',#37206,#8995);
#6840=LINE('',#37208,#8996);
#6841=LINE('',#37210,#8997);
#6842=LINE('',#37212,#8998);
#6843=LINE('',#37214,#8999);
#6844=LINE('',#37215,#9000);
#6845=LINE('',#37218,#9001);
#6846=LINE('',#37227,#9002);
#6847=LINE('',#37235,#9003);
#6848=LINE('',#37238,#9004);
#6849=LINE('',#37242,#9005);
#6850=LINE('',#37246,#9006);
#6851=LINE('',#37250,#9007);
#6852=LINE('',#37254,#9008);
#6853=LINE('',#37256,#9009);
#6854=LINE('',#37257,#9010);
#6855=LINE('',#37260,#9011);
#6856=LINE('',#37262,#9012);
#6857=LINE('',#37263,#9013);
#6858=LINE('',#37268,#9014);
#6859=LINE('',#37272,#9015);
#6860=LINE('',#37471,#9016);
#6861=LINE('',#37578,#9017);
#6862=LINE('',#37581,#9018);
#6863=LINE('',#37627,#9019);
#6864=LINE('',#37653,#9020);
#6865=LINE('',#37656,#9021);
#6866=LINE('',#37660,#9022);
#6867=LINE('',#37662,#9023);
#6868=LINE('',#37664,#9024);
#6869=LINE('',#37665,#9025);
#6870=LINE('',#37668,#9026);
#6871=LINE('',#37670,#9027);
#6872=LINE('',#37671,#9028);
#6873=LINE('',#37676,#9029);
#6874=LINE('',#37810,#9030);
#6875=LINE('',#37943,#9031);
#6876=LINE('',#37970,#9032);
#6877=LINE('',#37978,#9033);
#6878=LINE('',#37980,#9034);
#6879=LINE('',#37981,#9035);
#6880=LINE('',#37984,#9036);
#6881=LINE('',#37986,#9037);
#6882=LINE('',#37987,#9038);
#6883=LINE('',#37991,#9039);
#6884=LINE('',#37993,#9040);
#6885=LINE('',#37994,#9041);
#6886=LINE('',#37997,#9042);
#6887=LINE('',#37999,#9043);
#6888=LINE('',#38000,#9044);
#6889=LINE('',#38004,#9045);
#6890=LINE('',#38006,#9046);
#6891=LINE('',#38007,#9047);
#6892=LINE('',#38011,#9048);
#6893=LINE('',#38012,#9049);
#6894=LINE('',#38013,#9050);
#6895=LINE('',#38017,#9051);
#6896=LINE('',#38023,#9052);
#6897=LINE('',#38024,#9053);
#6898=LINE('',#38025,#9054);
#6899=LINE('',#38029,#9055);
#6900=LINE('',#38033,#9056);
#6901=LINE('',#38034,#9057);
#6902=LINE('',#38037,#9058);
#6903=LINE('',#38039,#9059);
#6904=LINE('',#38040,#9060);
#6905=LINE('',#38042,#9061);
#6906=LINE('',#38043,#9062);
#6907=LINE('',#38045,#9063);
#6908=LINE('',#38046,#9064);
#6909=LINE('',#38048,#9065);
#6910=LINE('',#38049,#9066);
#6911=LINE('',#38053,#9067);
#6912=LINE('',#38056,#9068);
#6913=LINE('',#38104,#9069);
#6914=LINE('',#38132,#9070);
#6915=LINE('',#38134,#9071);
#6916=LINE('',#38135,#9072);
#6917=LINE('',#38138,#9073);
#6918=LINE('',#38198,#9074);
#6919=LINE('',#38200,#9075);
#6920=LINE('',#38202,#9076);
#6921=LINE('',#38204,#9077);
#6922=LINE('',#38206,#9078);
#6923=LINE('',#38210,#9079);
#6924=LINE('',#38212,#9080);
#6925=LINE('',#38213,#9081);
#6926=LINE('',#38216,#9082);
#6927=LINE('',#38220,#9083);
#6928=LINE('',#38221,#9084);
#6929=LINE('',#38224,#9085);
#6930=LINE('',#38226,#9086);
#6931=LINE('',#38231,#9087);
#6932=LINE('',#38235,#9088);
#6933=LINE('',#38239,#9089);
#6934=LINE('',#38243,#9090);
#6935=LINE('',#38247,#9091);
#6936=LINE('',#38249,#9092);
#6937=LINE('',#38250,#9093);
#6938=LINE('',#38253,#9094);
#6939=LINE('',#38257,#9095);
#6940=LINE('',#38258,#9096);
#6941=LINE('',#38263,#9097);
#6942=LINE('',#38266,#9098);
#6943=LINE('',#38269,#9099);
#6944=LINE('',#38270,#9100);
#6945=LINE('',#38273,#9101);
#6946=LINE('',#38275,#9102);
#6947=LINE('',#38276,#9103);
#6948=LINE('',#38279,#9104);
#6949=LINE('',#38283,#9105);
#6950=LINE('',#38284,#9106);
#6951=LINE('',#38289,#9107);
#6952=LINE('',#38292,#9108);
#6953=LINE('',#38295,#9109);
#6954=LINE('',#38296,#9110);
#6955=LINE('',#38299,#9111);
#6956=LINE('',#38301,#9112);
#6957=LINE('',#38302,#9113);
#6958=LINE('',#38305,#9114);
#6959=LINE('',#38309,#9115);
#6960=LINE('',#38310,#9116);
#6961=LINE('',#38315,#9117);
#6962=LINE('',#38318,#9118);
#6963=LINE('',#38321,#9119);
#6964=LINE('',#38322,#9120);
#6965=LINE('',#38325,#9121);
#6966=LINE('',#38327,#9122);
#6967=LINE('',#38328,#9123);
#6968=LINE('',#38331,#9124);
#6969=LINE('',#38335,#9125);
#6970=LINE('',#38336,#9126);
#6971=LINE('',#38341,#9127);
#6972=LINE('',#38344,#9128);
#6973=LINE('',#38347,#9129);
#6974=LINE('',#38348,#9130);
#6975=LINE('',#38353,#9131);
#6976=LINE('',#38361,#9132);
#6977=LINE('',#38366,#9133);
#6978=LINE('',#38372,#9134);
#6979=LINE('',#38375,#9135);
#6980=LINE('',#38377,#9136);
#6981=LINE('',#38378,#9137);
#6982=LINE('',#38382,#9138);
#6983=LINE('',#38387,#9139);
#6984=LINE('',#38388,#9140);
#6985=LINE('',#38389,#9141);
#6986=LINE('',#38393,#9142);
#6987=LINE('',#38402,#9143);
#6988=LINE('',#38404,#9144);
#6989=LINE('',#38406,#9145);
#6990=LINE('',#38408,#9146);
#6991=LINE('',#38410,#9147);
#6992=LINE('',#38412,#9148);
#6993=LINE('',#38414,#9149);
#6994=LINE('',#38415,#9150);
#6995=LINE('',#38417,#9151);
#6996=LINE('',#38419,#9152);
#6997=LINE('',#38421,#9153);
#6998=LINE('',#38430,#9154);
#6999=LINE('',#38434,#9155);
#7000=LINE('',#38438,#9156);
#7001=LINE('',#38442,#9157);
#7002=LINE('',#38446,#9158);
#7003=LINE('',#38450,#9159);
#7004=LINE('',#38454,#9160);
#7005=LINE('',#38458,#9161);
#7006=LINE('',#38462,#9162);
#7007=LINE('',#38465,#9163);
#7008=LINE('',#38466,#9164);
#7009=LINE('',#38469,#9165);
#7010=LINE('',#38472,#9166);
#7011=LINE('',#38473,#9167);
#7012=LINE('',#38476,#9168);
#7013=LINE('',#38478,#9169);
#7014=LINE('',#38479,#9170);
#7015=LINE('',#38482,#9171);
#7016=LINE('',#38485,#9172);
#7017=LINE('',#38486,#9173);
#7018=LINE('',#38489,#9174);
#7019=LINE('',#38491,#9175);
#7020=LINE('',#38492,#9176);
#7021=LINE('',#38495,#9177);
#7022=LINE('',#38498,#9178);
#7023=LINE('',#38499,#9179);
#7024=LINE('',#38502,#9180);
#7025=LINE('',#38758,#9181);
#7026=LINE('',#38768,#9182);
#7027=LINE('',#38770,#9183);
#7028=LINE('',#38774,#9184);
#7029=LINE('',#38775,#9185);
#7030=LINE('',#38778,#9186);
#7031=LINE('',#38782,#9187);
#7032=LINE('',#38783,#9188);
#7033=LINE('',#38785,#9189);
#7034=LINE('',#38788,#9190);
#7035=LINE('',#38790,#9191);
#7036=LINE('',#38861,#9192);
#7037=LINE('',#38881,#9193);
#7038=LINE('',#38883,#9194);
#7039=LINE('',#38885,#9195);
#7040=LINE('',#38887,#9196);
#7041=LINE('',#38890,#9197);
#7042=LINE('',#38892,#9198);
#7043=LINE('',#38901,#9199);
#7044=LINE('',#38985,#9200);
#7045=LINE('',#39008,#9201);
#7046=LINE('',#39079,#9202);
#7047=LINE('',#39080,#9203);
#7048=LINE('',#39083,#9204);
#7049=LINE('',#39086,#9205);
#7050=LINE('',#39089,#9206);
#7051=LINE('',#39091,#9207);
#7052=LINE('',#39144,#9208);
#7053=LINE('',#39157,#9209);
#7054=LINE('',#39207,#9210);
#7055=LINE('',#39312,#9211);
#7056=LINE('',#39331,#9212);
#7057=LINE('',#39334,#9213);
#7058=LINE('',#39337,#9214);
#7059=LINE('',#39340,#9215);
#7060=LINE('',#39346,#9216);
#7061=LINE('',#39424,#9217);
#7062=LINE('',#39430,#9218);
#7063=LINE('',#39434,#9219);
#8986=VECTOR('',#30061,1.69267766952967);
#8987=VECTOR('',#30068,1.75);
#8988=VECTOR('',#30079,1.78232233047033);
#8989=VECTOR('',#30086,1.8);
#8990=VECTOR('',#30091,0.330000000000001);
#8991=VECTOR('',#30104,5.4);
#8992=VECTOR('',#30119,0.305);
#8993=VECTOR('',#30124,0.329999999999999);
#8994=VECTOR('',#30133,0.305);
#8995=VECTOR('',#30136,1.);
#8996=VECTOR('',#30137,1.);
#8997=VECTOR('',#30138,1.);
#8998=VECTOR('',#30139,1.);
#8999=VECTOR('',#30140,1.);
#9000=VECTOR('',#30141,1.);
#9001=VECTOR('',#30144,1.);
#9002=VECTOR('',#30147,1.);
#9003=VECTOR('',#30150,1.);
#9004=VECTOR('',#30151,1.);
#9005=VECTOR('',#30154,1.);
#9006=VECTOR('',#30157,1.);
#9007=VECTOR('',#30160,1.);
#9008=VECTOR('',#30165,1.);
#9009=VECTOR('',#30166,1.);
#9010=VECTOR('',#30167,1.);
#9011=VECTOR('',#30170,1.);
#9012=VECTOR('',#30171,1.);
#9013=VECTOR('',#30172,1.);
#9014=VECTOR('',#30177,5.29267766952966);
#9015=VECTOR('',#30182,5.4);
#9016=VECTOR('',#30189,1.);
#9017=VECTOR('',#30196,5.5);
#9018=VECTOR('',#30197,1.);
#9019=VECTOR('',#30198,1.);
#9020=VECTOR('',#30203,0.700000000000003);
#9021=VECTOR('',#30208,5.48232233047034);
#9022=VECTOR('',#30211,1.);
#9023=VECTOR('',#30212,1.);
#9024=VECTOR('',#30213,1.);
#9025=VECTOR('',#30214,1.);
#9026=VECTOR('',#30217,1.);
#9027=VECTOR('',#30218,1.);
#9028=VECTOR('',#30219,1.);
#9029=VECTOR('',#30224,1.);
#9030=VECTOR('',#30227,1.);
#9031=VECTOR('',#30228,1.);
#9032=VECTOR('',#30229,1.);
#9033=VECTOR('',#30232,1.);
#9034=VECTOR('',#30233,1.);
#9035=VECTOR('',#30234,1.);
#9036=VECTOR('',#30237,1.);
#9037=VECTOR('',#30238,1.);
#9038=VECTOR('',#30239,1.);
#9039=VECTOR('',#30242,1.);
#9040=VECTOR('',#30243,1.);
#9041=VECTOR('',#30244,1.);
#9042=VECTOR('',#30247,1.);
#9043=VECTOR('',#30248,1.);
#9044=VECTOR('',#30249,1.);
#9045=VECTOR('',#30252,1.);
#9046=VECTOR('',#30253,1.);
#9047=VECTOR('',#30254,1.);
#9048=VECTOR('',#30257,1.);
#9049=VECTOR('',#30258,1.);
#9050=VECTOR('',#30259,1.);
#9051=VECTOR('',#30262,1.);
#9052=VECTOR('',#30269,1.);
#9053=VECTOR('',#30270,1.);
#9054=VECTOR('',#30271,1.);
#9055=VECTOR('',#30274,1.);
#9056=VECTOR('',#30281,1.);
#9057=VECTOR('',#30282,1.);
#9058=VECTOR('',#30285,1.);
#9059=VECTOR('',#30286,1.);
#9060=VECTOR('',#30287,1.);
#9061=VECTOR('',#30290,1.);
#9062=VECTOR('',#30291,1.);
#9063=VECTOR('',#30294,1.);
#9064=VECTOR('',#30295,1.);
#9065=VECTOR('',#30298,1.);
#9066=VECTOR('',#30299,1.);
#9067=VECTOR('',#30304,1.);
#9068=VECTOR('',#30307,1.);
#9069=VECTOR('',#30310,1.);
#9070=VECTOR('',#30313,1.);
#9071=VECTOR('',#30314,1.);
#9072=VECTOR('',#30315,1.);
#9073=VECTOR('',#30318,1.);
#9074=VECTOR('',#30323,1.);
#9075=VECTOR('',#30324,1.);
#9076=VECTOR('',#30325,1.);
#9077=VECTOR('',#30326,1.);
#9078=VECTOR('',#30327,1.);
#9079=VECTOR('',#30330,1.);
#9080=VECTOR('',#30331,1.);
#9081=VECTOR('',#30332,1.);
#9082=VECTOR('',#30333,1.);
#9083=VECTOR('',#30336,1.);
#9084=VECTOR('',#30337,1.);
#9085=VECTOR('',#30342,1.);
#9086=VECTOR('',#30345,1.);
#9087=VECTOR('',#30350,1.);
#9088=VECTOR('',#30353,1.);
#9089=VECTOR('',#30356,1.);
#9090=VECTOR('',#30359,1.);
#9091=VECTOR('',#30364,1.);
#9092=VECTOR('',#30365,1.);
#9093=VECTOR('',#30366,1.);
#9094=VECTOR('',#30369,1.);
#9095=VECTOR('',#30374,1.);
#9096=VECTOR('',#30375,1.);
#9097=VECTOR('',#30382,1.);
#9098=VECTOR('',#30385,1.);
#9099=VECTOR('',#30388,1.);
#9100=VECTOR('',#30389,1.);
#9101=VECTOR('',#30392,1.);
#9102=VECTOR('',#30393,1.);
#9103=VECTOR('',#30394,1.);
#9104=VECTOR('',#30397,1.);
#9105=VECTOR('',#30402,1.);
#9106=VECTOR('',#30403,1.);
#9107=VECTOR('',#30410,1.);
#9108=VECTOR('',#30413,1.);
#9109=VECTOR('',#30416,1.);
#9110=VECTOR('',#30417,1.);
#9111=VECTOR('',#30420,1.);
#9112=VECTOR('',#30421,1.);
#9113=VECTOR('',#30422,1.);
#9114=VECTOR('',#30425,1.);
#9115=VECTOR('',#30430,1.);
#9116=VECTOR('',#30431,1.);
#9117=VECTOR('',#30438,1.);
#9118=VECTOR('',#30441,1.);
#9119=VECTOR('',#30444,1.);
#9120=VECTOR('',#30445,1.);
#9121=VECTOR('',#30448,1.);
#9122=VECTOR('',#30449,1.);
#9123=VECTOR('',#30450,1.);
#9124=VECTOR('',#30453,1.);
#9125=VECTOR('',#30458,1.);
#9126=VECTOR('',#30459,1.);
#9127=VECTOR('',#30466,1.);
#9128=VECTOR('',#30469,1.);
#9129=VECTOR('',#30472,1.);
#9130=VECTOR('',#30473,1.);
#9131=VECTOR('',#30478,0.330000000000001);
#9132=VECTOR('',#30489,0.305);
#9133=VECTOR('',#30494,0.33);
#9134=VECTOR('',#30503,0.305);
#9135=VECTOR('',#30506,1.);
#9136=VECTOR('',#30507,1.);
#9137=VECTOR('',#30508,1.);
#9138=VECTOR('',#30511,1.);
#9139=VECTOR('',#30518,1.);
#9140=VECTOR('',#30519,1.);
#9141=VECTOR('',#30520,1.);
#9142=VECTOR('',#30527,1.);
#9143=VECTOR('',#30530,1.);
#9144=VECTOR('',#30531,1.);
#9145=VECTOR('',#30532,1.);
#9146=VECTOR('',#30533,1.);
#9147=VECTOR('',#30534,1.);
#9148=VECTOR('',#30535,1.);
#9149=VECTOR('',#30536,1.);
#9150=VECTOR('',#30537,1.);
#9151=VECTOR('',#30538,1.);
#9152=VECTOR('',#30539,1.);
#9153=VECTOR('',#30540,1.);
#9154=VECTOR('',#30543,1.);
#9155=VECTOR('',#30546,1.);
#9156=VECTOR('',#30549,1.);
#9157=VECTOR('',#30552,1.);
#9158=VECTOR('',#30555,1.);
#9159=VECTOR('',#30558,1.);
#9160=VECTOR('',#30561,1.);
#9161=VECTOR('',#30564,1.);
#9162=VECTOR('',#30567,1.);
#9163=VECTOR('',#30572,1.);
#9164=VECTOR('',#30573,1.);
#9165=VECTOR('',#30576,1.);
#9166=VECTOR('',#30581,1.);
#9167=VECTOR('',#30582,1.);
#9168=VECTOR('',#30587,1.);
#9169=VECTOR('',#30590,1.);
#9170=VECTOR('',#30591,1.);
#9171=VECTOR('',#30594,1.);
#9172=VECTOR('',#30599,1.);
#9173=VECTOR('',#30600,1.);
#9174=VECTOR('',#30605,1.);
#9175=VECTOR('',#30608,1.);
#9176=VECTOR('',#30609,1.);
#9177=VECTOR('',#30612,1.);
#9178=VECTOR('',#30617,1.);
#9179=VECTOR('',#30618,1.);
#9180=VECTOR('',#30623,1.);
#9181=VECTOR('',#30624,1.);
#9182=VECTOR('',#30627,1.);
#9183=VECTOR('',#30628,1.);
#9184=VECTOR('',#30633,1.);
#9185=VECTOR('',#30634,1.);
#9186=VECTOR('',#30637,1.);
#9187=VECTOR('',#30642,1.);
#9188=VECTOR('',#30643,1.);
#9189=VECTOR('',#30646,1.);
#9190=VECTOR('',#30651,1.);
#9191=VECTOR('',#30654,1.);
#9192=VECTOR('',#30655,1.);
#9193=VECTOR('',#30662,1.);
#9194=VECTOR('',#30665,1.);
#9195=VECTOR('',#30668,1.);
#9196=VECTOR('',#30671,1.);
#9197=VECTOR('',#30674,1.);
#9198=VECTOR('',#30675,1.);
#9199=VECTOR('',#30680,1.);
#9200=VECTOR('',#30683,1.);
#9201=VECTOR('',#30684,1.);
#9202=VECTOR('',#30687,1.);
#9203=VECTOR('',#30688,1.);
#9204=VECTOR('',#30691,1.);
#9205=VECTOR('',#30696,1.);
#9206=VECTOR('',#30699,1.);
#9207=VECTOR('',#30700,1.);
#9208=VECTOR('',#30705,1.);
#9209=VECTOR('',#30712,1.);
#9210=VECTOR('',#30715,1.);
#9211=VECTOR('',#30726,1.);
#9212=VECTOR('',#30761,0.1525);
#9213=VECTOR('',#30764,0.1525);
#9214=VECTOR('',#30767,0.1525);
#9215=VECTOR('',#30770,0.1525);
#9216=VECTOR('',#30777,0.405000000000001);
#9217=VECTOR('',#30780,1.005);
#9218=VECTOR('',#30789,0.605000000000004);
#9219=VECTOR('',#30794,3.5);
#11088=VERTEX_POINT('',#37041);
#11089=VERTEX_POINT('',#37043);
#11090=VERTEX_POINT('',#37045);
#11091=VERTEX_POINT('',#37049);
#11092=VERTEX_POINT('',#37051);
#11093=VERTEX_POINT('',#37055);
#11094=VERTEX_POINT('',#37058);
#11095=VERTEX_POINT('',#37060);
#11096=VERTEX_POINT('',#37064);
#11097=VERTEX_POINT('',#37066);
#11098=VERTEX_POINT('',#37136);
#11099=VERTEX_POINT('',#37137);
#11100=VERTEX_POINT('',#37144);
#11101=VERTEX_POINT('',#37146);
#11102=VERTEX_POINT('',#37148);
#11103=VERTEX_POINT('',#37153);
#11104=VERTEX_POINT('',#37154);
#11105=VERTEX_POINT('',#37157);
#11106=VERTEX_POINT('',#37160);
#11107=VERTEX_POINT('',#37162);
#11108=VERTEX_POINT('',#37169);
#11109=VERTEX_POINT('',#37171);
#11110=VERTEX_POINT('',#37178);
#11111=VERTEX_POINT('',#37180);
#11112=VERTEX_POINT('',#37189);
#11113=VERTEX_POINT('',#37193);
#11114=VERTEX_POINT('',#37195);
#11115=VERTEX_POINT('',#37200);
#11116=VERTEX_POINT('',#37204);
#11117=VERTEX_POINT('',#37205);
#11118=VERTEX_POINT('',#37207);
#11119=VERTEX_POINT('',#37209);
#11120=VERTEX_POINT('',#37211);
#11121=VERTEX_POINT('',#37213);
#11122=VERTEX_POINT('',#37217);
#11123=VERTEX_POINT('',#37219);
#11124=VERTEX_POINT('',#37221);
#11125=VERTEX_POINT('',#37226);
#11126=VERTEX_POINT('',#37228);
#11127=VERTEX_POINT('',#37233);
#11128=VERTEX_POINT('',#37236);
#11129=VERTEX_POINT('',#37237);
#11130=VERTEX_POINT('',#37239);
#11131=VERTEX_POINT('',#37241);
#11132=VERTEX_POINT('',#37244);
#11133=VERTEX_POINT('',#37245);
#11134=VERTEX_POINT('',#37247);
#11135=VERTEX_POINT('',#37249);
#11136=VERTEX_POINT('',#37253);
#11137=VERTEX_POINT('',#37255);
#11138=VERTEX_POINT('',#37259);
#11139=VERTEX_POINT('',#37261);
#11140=VERTEX_POINT('',#37265);
#11141=VERTEX_POINT('',#37267);
#11142=VERTEX_POINT('',#37271);
#11143=VERTEX_POINT('',#37275);
#11144=VERTEX_POINT('',#37469);
#11145=VERTEX_POINT('',#37470);
#11146=VERTEX_POINT('',#37472);
#11147=VERTEX_POINT('',#37574);
#11148=VERTEX_POINT('',#37575);
#11149=VERTEX_POINT('',#37579);
#11150=VERTEX_POINT('',#37580);
#11151=VERTEX_POINT('',#37582);
#11152=VERTEX_POINT('',#37590);
#11153=VERTEX_POINT('',#37618);
#11154=VERTEX_POINT('',#37626);
#11155=VERTEX_POINT('',#37628);
#11156=VERTEX_POINT('',#37639);
#11157=VERTEX_POINT('',#37652);
#11158=VERTEX_POINT('',#37658);
#11159=VERTEX_POINT('',#37659);
#11160=VERTEX_POINT('',#37661);
#11161=VERTEX_POINT('',#37663);
#11162=VERTEX_POINT('',#37667);
#11163=VERTEX_POINT('',#37669);
#11164=VERTEX_POINT('',#37673);
#11165=VERTEX_POINT('',#37675);
#11166=VERTEX_POINT('',#37710);
#11167=VERTEX_POINT('',#37711);
#11168=VERTEX_POINT('',#37752);
#11169=VERTEX_POINT('',#37757);
#11170=VERTEX_POINT('',#37843);
#11171=VERTEX_POINT('',#37844);
#11172=VERTEX_POINT('',#37897);
#11173=VERTEX_POINT('',#37902);
#11174=VERTEX_POINT('',#37969);
#11175=VERTEX_POINT('',#37977);
#11176=VERTEX_POINT('',#37979);
#11177=VERTEX_POINT('',#37983);
#11178=VERTEX_POINT('',#37985);
#11179=VERTEX_POINT('',#37989);
#11180=VERTEX_POINT('',#37990);
#11181=VERTEX_POINT('',#37992);
#11182=VERTEX_POINT('',#37996);
#11183=VERTEX_POINT('',#37998);
#11184=VERTEX_POINT('',#38002);
#11185=VERTEX_POINT('',#38003);
#11186=VERTEX_POINT('',#38005);
#11187=VERTEX_POINT('',#38009);
#11188=VERTEX_POINT('',#38010);
#11189=VERTEX_POINT('',#38015);
#11190=VERTEX_POINT('',#38016);
#11191=VERTEX_POINT('',#38021);
#11192=VERTEX_POINT('',#38022);
#11193=VERTEX_POINT('',#38027);
#11194=VERTEX_POINT('',#38028);
#11195=VERTEX_POINT('',#38036);
#11196=VERTEX_POINT('',#38038);
#11197=VERTEX_POINT('',#38051);
#11198=VERTEX_POINT('',#38055);
#11199=VERTEX_POINT('',#38098);
#11200=VERTEX_POINT('',#38131);
#11201=VERTEX_POINT('',#38133);
#11202=VERTEX_POINT('',#38137);
#11203=VERTEX_POINT('',#38139);
#11204=VERTEX_POINT('',#38180);
#11205=VERTEX_POINT('',#38191);
#11206=VERTEX_POINT('',#38199);
#11207=VERTEX_POINT('',#38201);
#11208=VERTEX_POINT('',#38203);
#11209=VERTEX_POINT('',#38205);
#11210=VERTEX_POINT('',#38207);
#11211=VERTEX_POINT('',#38209);
#11212=VERTEX_POINT('',#38211);
#11213=VERTEX_POINT('',#38214);
#11214=VERTEX_POINT('',#38215);
#11215=VERTEX_POINT('',#38217);
#11216=VERTEX_POINT('',#38219);
#11217=VERTEX_POINT('',#38229);
#11218=VERTEX_POINT('',#38230);
#11219=VERTEX_POINT('',#38232);
#11220=VERTEX_POINT('',#38234);
#11221=VERTEX_POINT('',#38237);
#11222=VERTEX_POINT('',#38238);
#11223=VERTEX_POINT('',#38240);
#11224=VERTEX_POINT('',#38242);
#11225=VERTEX_POINT('',#38246);
#11226=VERTEX_POINT('',#38248);
#11227=VERTEX_POINT('',#38252);
#11228=VERTEX_POINT('',#38256);
#11229=VERTEX_POINT('',#38262);
#11230=VERTEX_POINT('',#38264);
#11231=VERTEX_POINT('',#38268);
#11232=VERTEX_POINT('',#38272);
#11233=VERTEX_POINT('',#38274);
#11234=VERTEX_POINT('',#38278);
#11235=VERTEX_POINT('',#38282);
#11236=VERTEX_POINT('',#38288);
#11237=VERTEX_POINT('',#38290);
#11238=VERTEX_POINT('',#38294);
#11239=VERTEX_POINT('',#38298);
#11240=VERTEX_POINT('',#38300);
#11241=VERTEX_POINT('',#38304);
#11242=VERTEX_POINT('',#38308);
#11243=VERTEX_POINT('',#38314);
#11244=VERTEX_POINT('',#38316);
#11245=VERTEX_POINT('',#38320);
#11246=VERTEX_POINT('',#38324);
#11247=VERTEX_POINT('',#38326);
#11248=VERTEX_POINT('',#38330);
#11249=VERTEX_POINT('',#38334);
#11250=VERTEX_POINT('',#38340);
#11251=VERTEX_POINT('',#38342);
#11252=VERTEX_POINT('',#38346);
#11253=VERTEX_POINT('',#38350);
#11254=VERTEX_POINT('',#38352);
#11255=VERTEX_POINT('',#38354);
#11256=VERTEX_POINT('',#38359);
#11257=VERTEX_POINT('',#38363);
#11258=VERTEX_POINT('',#38365);
#11259=VERTEX_POINT('',#38370);
#11260=VERTEX_POINT('',#38374);
#11261=VERTEX_POINT('',#38376);
#11262=VERTEX_POINT('',#38380);
#11263=VERTEX_POINT('',#38381);
#11264=VERTEX_POINT('',#38386);
#11265=VERTEX_POINT('',#38395);
#11266=VERTEX_POINT('',#38396);
#11267=VERTEX_POINT('',#38401);
#11268=VERTEX_POINT('',#38403);
#11269=VERTEX_POINT('',#38405);
#11270=VERTEX_POINT('',#38407);
#11271=VERTEX_POINT('',#38409);
#11272=VERTEX_POINT('',#38411);
#11273=VERTEX_POINT('',#38413);
#11274=VERTEX_POINT('',#38416);
#11275=VERTEX_POINT('',#38418);
#11276=VERTEX_POINT('',#38420);
#11277=VERTEX_POINT('',#38422);
#11278=VERTEX_POINT('',#38427);
#11279=VERTEX_POINT('',#38429);
#11280=VERTEX_POINT('',#38431);
#11281=VERTEX_POINT('',#38433);
#11282=VERTEX_POINT('',#38435);
#11283=VERTEX_POINT('',#38437);
#11284=VERTEX_POINT('',#38440);
#11285=VERTEX_POINT('',#38441);
#11286=VERTEX_POINT('',#38443);
#11287=VERTEX_POINT('',#38445);
#11288=VERTEX_POINT('',#38448);
#11289=VERTEX_POINT('',#38449);
#11290=VERTEX_POINT('',#38451);
#11291=VERTEX_POINT('',#38453);
#11292=VERTEX_POINT('',#38456);
#11293=VERTEX_POINT('',#38457);
#11294=VERTEX_POINT('',#38459);
#11295=VERTEX_POINT('',#38461);
#11296=VERTEX_POINT('',#38468);
#11297=VERTEX_POINT('',#38481);
#11298=VERTEX_POINT('',#38494);
#11299=VERTEX_POINT('',#38535);
#11300=VERTEX_POINT('',#38624);
#11301=VERTEX_POINT('',#38665);
#11302=VERTEX_POINT('',#38750);
#11303=VERTEX_POINT('',#38767);
#11304=VERTEX_POINT('',#38769);
#11305=VERTEX_POINT('',#38773);
#11306=VERTEX_POINT('',#38777);
#11307=VERTEX_POINT('',#38781);
#11308=VERTEX_POINT('',#38889);
#11309=VERTEX_POINT('',#38891);
#11310=VERTEX_POINT('',#38898);
#11311=VERTEX_POINT('',#38900);
#11312=VERTEX_POINT('',#38983);
#11313=VERTEX_POINT('',#38984);
#11314=VERTEX_POINT('',#38986);
#11315=VERTEX_POINT('',#39007);
#11316=VERTEX_POINT('',#39078);
#11317=VERTEX_POINT('',#39082);
#11318=VERTEX_POINT('',#39088);
#11319=VERTEX_POINT('',#39090);
#11320=VERTEX_POINT('',#39092);
#11321=VERTEX_POINT('',#39146);
#11322=VERTEX_POINT('',#39156);
#11323=VERTEX_POINT('',#39201);
#11324=VERTEX_POINT('',#39299);
#11325=VERTEX_POINT('',#39330);
#11326=VERTEX_POINT('',#39333);
#11327=VERTEX_POINT('',#39336);
#11328=VERTEX_POINT('',#39339);
#11329=VERTEX_POINT('',#39342);
#11330=VERTEX_POINT('',#39345);
#11331=VERTEX_POINT('',#39347);
#11332=VERTEX_POINT('',#39385);
#11333=VERTEX_POINT('',#39386);
#11334=VERTEX_POINT('',#39423);
#11335=VERTEX_POINT('',#39427);
#11336=VERTEX_POINT('',#39432);
#13641=EDGE_CURVE('',#11088,#11088,#5815,.T.);
#13642=EDGE_CURVE('',#11088,#11089,#6830,.T.);
#13643=EDGE_CURVE('',#11089,#11090,#5816,.T.);
#13644=EDGE_CURVE('',#11090,#11089,#5817,.T.);
#13645=EDGE_CURVE('',#11090,#11091,#6831,.T.);
#13646=EDGE_CURVE('',#11092,#11091,#5818,.T.);
#13647=EDGE_CURVE('',#11091,#11092,#5819,.T.);
#13648=EDGE_CURVE('',#11093,#11093,#5820,.T.);
#13649=EDGE_CURVE('',#11092,#11094,#6832,.T.);
#13650=EDGE_CURVE('',#11094,#11095,#5821,.T.);
#13651=EDGE_CURVE('',#11095,#11094,#5822,.T.);
#13652=EDGE_CURVE('',#11095,#11096,#6833,.T.);
#13653=EDGE_CURVE('',#11097,#11096,#174,.T.);
#13654=EDGE_CURVE('',#11096,#11097,#175,.T.);
#13655=EDGE_CURVE('',#11098,#11099,#176,.T.);
#13656=EDGE_CURVE('',#11099,#11100,#5823,.T.);
#13657=EDGE_CURVE('',#11100,#11101,#6834,.T.);
#13658=EDGE_CURVE('',#11101,#11102,#5824,.T.);
#13659=EDGE_CURVE('',#11102,#11101,#5825,.T.);
#13660=EDGE_CURVE('',#11100,#11098,#5826,.T.);
#13661=EDGE_CURVE('',#11103,#11104,#5827,.T.);
#13662=EDGE_CURVE('',#11104,#11103,#5828,.T.);
#13663=EDGE_CURVE('',#11103,#11105,#6835,.T.);
#13664=EDGE_CURVE('',#11105,#11099,#5829,.T.);
#13665=EDGE_CURVE('',#11098,#11106,#5830,.T.);
#13666=EDGE_CURVE('',#11107,#11106,#177,.T.);
#13667=EDGE_CURVE('',#11107,#11108,#5831,.T.);
#13668=EDGE_CURVE('',#11109,#11108,#178,.T.);
#13669=EDGE_CURVE('',#11109,#11110,#5832,.T.);
#13670=EDGE_CURVE('',#11111,#11110,#179,.T.);
#13671=EDGE_CURVE('',#11111,#11105,#5833,.T.);
#13672=EDGE_CURVE('',#11112,#11112,#5834,.T.);
#13673=EDGE_CURVE('',#11112,#11102,#6836,.T.);
#13674=EDGE_CURVE('',#11110,#11113,#5835,.T.);
#13675=EDGE_CURVE('',#11113,#11114,#6837,.T.);
#13676=EDGE_CURVE('',#11114,#11114,#5836,.T.);
#13677=EDGE_CURVE('',#11113,#11111,#5837,.T.);
#13678=EDGE_CURVE('',#11115,#11115,#5838,.T.);
#13679=EDGE_CURVE('',#11115,#11114,#6838,.T.);
#13680=EDGE_CURVE('',#11116,#11117,#6839,.T.);
#13681=EDGE_CURVE('',#11117,#11118,#6840,.T.);
#13682=EDGE_CURVE('',#11118,#11119,#6841,.T.);
#13683=EDGE_CURVE('',#11119,#11120,#6842,.T.);
#13684=EDGE_CURVE('',#11120,#11121,#6843,.T.);
#13685=EDGE_CURVE('',#11121,#11116,#6844,.T.);
#13686=EDGE_CURVE('',#11122,#11117,#6845,.T.);
#13687=EDGE_CURVE('',#11123,#11122,#5839,.T.);
#13688=EDGE_CURVE('',#11124,#11123,#180,.T.);
#13689=EDGE_CURVE('',#11125,#11124,#6846,.T.);
#13690=EDGE_CURVE('',#11126,#11125,#181,.T.);
#13691=EDGE_CURVE('',#11127,#11126,#5840,.T.);
#13692=EDGE_CURVE('',#11118,#11127,#6847,.T.);
#13693=EDGE_CURVE('',#11128,#11129,#6848,.T.);
#13694=EDGE_CURVE('',#11130,#11128,#5841,.T.);
#13695=EDGE_CURVE('',#11131,#11130,#6849,.T.);
#13696=EDGE_CURVE('',#11129,#11131,#5842,.T.);
#13697=EDGE_CURVE('',#11132,#11133,#6850,.T.);
#13698=EDGE_CURVE('',#11134,#11132,#5843,.T.);
#13699=EDGE_CURVE('',#11135,#11134,#6851,.T.);
#13700=EDGE_CURVE('',#11133,#11135,#5844,.T.);
#13701=EDGE_CURVE('',#11136,#11116,#6852,.T.);
#13702=EDGE_CURVE('',#11136,#11137,#6853,.T.);
#13703=EDGE_CURVE('',#11137,#11122,#6854,.T.);
#13704=EDGE_CURVE('',#11121,#11138,#6855,.T.);
#13705=EDGE_CURVE('',#11138,#11139,#6856,.T.);
#13706=EDGE_CURVE('',#11139,#11136,#6857,.T.);
#13707=EDGE_CURVE('',#11140,#11140,#5845,.T.);
#13708=EDGE_CURVE('',#11140,#11141,#6858,.T.);
#13709=EDGE_CURVE('',#11141,#11141,#5846,.T.);
#13710=EDGE_CURVE('',#11140,#11142,#6859,.T.);
#13711=EDGE_CURVE('',#11142,#11142,#5847,.T.);
#13712=EDGE_CURVE('',#11143,#11143,#5848,.T.);
#13713=EDGE_CURVE('',#11144,#11145,#6860,.T.);
#13714=EDGE_CURVE('',#11145,#11146,#182,.T.);
#13715=EDGE_CURVE('',#11146,#11145,#183,.T.);
#13716=EDGE_CURVE('',#11144,#11144,#184,.T.);
#13717=EDGE_CURVE('',#11147,#11148,#5849,.T.);
#13718=EDGE_CURVE('',#11148,#11147,#5850,.T.);
#13719=EDGE_CURVE('',#11148,#11104,#6861,.T.);
#13720=EDGE_CURVE('',#11149,#11150,#6862,.T.);
#13721=EDGE_CURVE('',#11151,#11150,#185,.F.);
#13722=EDGE_CURVE('',#11151,#11152,#186,.T.);
#13723=EDGE_CURVE('',#11153,#11152,#187,.F.);
#13724=EDGE_CURVE('',#11153,#11154,#6863,.T.);
#13725=EDGE_CURVE('',#11155,#11154,#188,.F.);
#13726=EDGE_CURVE('',#11156,#11155,#5851,.T.);
#13727=EDGE_CURVE('',#11149,#11156,#189,.F.);
#13728=EDGE_CURVE('',#11146,#11157,#6864,.T.);
#13729=EDGE_CURVE('',#11157,#11157,#5852,.T.);
#13730=EDGE_CURVE('',#11142,#11147,#6865,.T.);
#13731=EDGE_CURVE('',#11158,#11159,#6866,.T.);
#13732=EDGE_CURVE('',#11159,#11160,#6867,.T.);
#13733=EDGE_CURVE('',#11160,#11161,#6868,.F.);
#13734=EDGE_CURVE('',#11161,#11158,#6869,.T.);
#13735=EDGE_CURVE('',#11159,#11162,#6870,.T.);
#13736=EDGE_CURVE('',#11163,#11162,#6871,.T.);
#13737=EDGE_CURVE('',#11163,#11160,#6872,.T.);
#13738=EDGE_CURVE('',#11158,#11164,#5853,.T.);
#13739=EDGE_CURVE('',#11164,#11165,#6873,.T.);
#13740=EDGE_CURVE('',#11165,#11159,#5854,.T.);
#13741=EDGE_CURVE('',#11166,#11167,#190,.T.);
#13742=EDGE_CURVE('',#11168,#11167,#191,.T.);
#13743=EDGE_CURVE('',#11168,#11169,#192,.T.);
#13744=EDGE_CURVE('',#11169,#11166,#6874,.T.);
#13745=EDGE_CURVE('',#11170,#11171,#193,.T.);
#13746=EDGE_CURVE('',#11172,#11171,#194,.T.);
#13747=EDGE_CURVE('',#11172,#11173,#195,.T.);
#13748=EDGE_CURVE('',#11173,#11170,#6875,.T.);
#13749=EDGE_CURVE('',#11171,#11124,#196,.T.);
#13750=EDGE_CURVE('',#11124,#11174,#6876,.T.);
#13751=EDGE_CURVE('',#11174,#11172,#197,.T.);
#13752=EDGE_CURVE('',#11127,#11175,#6877,.T.);
#13753=EDGE_CURVE('',#11175,#11176,#6878,.T.);
#13754=EDGE_CURVE('',#11176,#11119,#6879,.T.);
#13755=EDGE_CURVE('',#11176,#11177,#6880,.T.);
#13756=EDGE_CURVE('',#11177,#11178,#6881,.T.);
#13757=EDGE_CURVE('',#11178,#11120,#6882,.T.);
#13758=EDGE_CURVE('',#11179,#11180,#6883,.T.);
#13759=EDGE_CURVE('',#11181,#11179,#6884,.T.);
#13760=EDGE_CURVE('',#11180,#11181,#6885,.T.);
#13761=EDGE_CURVE('',#11182,#11181,#6886,.T.);
#13762=EDGE_CURVE('',#11179,#11183,#6887,.T.);
#13763=EDGE_CURVE('',#11183,#11182,#6888,.T.);
#13764=EDGE_CURVE('',#11184,#11185,#6889,.T.);
#13765=EDGE_CURVE('',#11186,#11184,#6890,.T.);
#13766=EDGE_CURVE('',#11185,#11186,#6891,.T.);
#13767=EDGE_CURVE('',#11187,#11188,#6892,.T.);
#13768=EDGE_CURVE('',#11188,#11186,#6893,.T.);
#13769=EDGE_CURVE('',#11184,#11187,#6894,.T.);
#13770=EDGE_CURVE('',#11189,#11190,#6895,.T.);
#13771=EDGE_CURVE('',#11190,#11188,#5855,.T.);
#13772=EDGE_CURVE('',#11187,#11189,#5856,.T.);
#13773=EDGE_CURVE('',#11191,#11192,#6896,.T.);
#13774=EDGE_CURVE('',#11192,#11190,#6897,.T.);
#13775=EDGE_CURVE('',#11189,#11191,#6898,.T.);
#13776=EDGE_CURVE('',#11193,#11194,#6899,.T.);
#13777=EDGE_CURVE('',#11194,#11192,#5857,.T.);
#13778=EDGE_CURVE('',#11191,#11193,#5858,.T.);
#13779=EDGE_CURVE('',#11193,#11180,#6900,.T.);
#13780=EDGE_CURVE('',#11181,#11194,#6901,.T.);
#13781=EDGE_CURVE('',#11195,#11185,#6902,.T.);
#13782=EDGE_CURVE('',#11186,#11196,#6903,.T.);
#13783=EDGE_CURVE('',#11196,#11195,#6904,.T.);
#13784=EDGE_CURVE('',#11180,#11184,#6905,.T.);
#13785=EDGE_CURVE('',#11185,#11179,#6906,.T.);
#13786=EDGE_CURVE('',#11138,#11195,#6907,.T.);
#13787=EDGE_CURVE('',#11196,#11139,#6908,.T.);
#13788=EDGE_CURVE('',#11177,#11182,#6909,.T.);
#13789=EDGE_CURVE('',#11183,#11178,#6910,.T.);
#13790=EDGE_CURVE('',#11137,#11197,#5859,.T.);
#13791=EDGE_CURVE('',#11197,#11123,#6911,.T.);
#13792=EDGE_CURVE('',#11126,#11198,#6912,.T.);
#13793=EDGE_CURVE('',#11198,#11175,#5860,.T.);
#13794=EDGE_CURVE('',#11197,#11174,#198,.T.);
#13795=EDGE_CURVE('',#11167,#11199,#199,.T.);
#13796=EDGE_CURVE('',#11199,#11125,#6913,.T.);
#13797=EDGE_CURVE('',#11125,#11168,#200,.T.);
#13798=EDGE_CURVE('',#11199,#11198,#201,.T.);
#13799=EDGE_CURVE('',#11175,#11200,#6914,.T.);
#13800=EDGE_CURVE('',#11201,#11200,#6915,.T.);
#13801=EDGE_CURVE('',#11194,#11201,#6916,.T.);
#13802=EDGE_CURVE('',#11166,#11202,#6917,.T.);
#13803=EDGE_CURVE('',#11203,#11202,#202,.T.);
#13804=EDGE_CURVE('',#11204,#11203,#203,.T.);
#13805=EDGE_CURVE('',#11205,#11204,#204,.T.);
#13806=EDGE_CURVE('',#11200,#11205,#5861,.T.);
#13807=EDGE_CURVE('',#11170,#11169,#6918,.T.);
#13808=EDGE_CURVE('',#11173,#11206,#6919,.T.);
#13809=EDGE_CURVE('',#11207,#11206,#6920,.T.);
#13810=EDGE_CURVE('',#11208,#11207,#6921,.T.);
#13811=EDGE_CURVE('',#11209,#11208,#6922,.T.);
#13812=EDGE_CURVE('',#11210,#11209,#5862,.T.);
#13813=EDGE_CURVE('',#11211,#11210,#6923,.T.);
#13814=EDGE_CURVE('',#11212,#11211,#6924,.T.);
#13815=EDGE_CURVE('',#11202,#11212,#6925,.T.);
#13816=EDGE_CURVE('',#11213,#11214,#6926,.T.);
#13817=EDGE_CURVE('',#11215,#11213,#5863,.T.);
#13818=EDGE_CURVE('',#11216,#11215,#6927,.T.);
#13819=EDGE_CURVE('',#11214,#11216,#6928,.T.);
#13820=EDGE_CURVE('',#11195,#11183,#6929,.T.);
#13821=EDGE_CURVE('',#11178,#11138,#6930,.T.);
#13822=EDGE_CURVE('',#11217,#11218,#6931,.T.);
#13823=EDGE_CURVE('',#11219,#11217,#5864,.T.);
#13824=EDGE_CURVE('',#11220,#11219,#6932,.T.);
#13825=EDGE_CURVE('',#11218,#11220,#5865,.T.);
#13826=EDGE_CURVE('',#11221,#11222,#6933,.T.);
#13827=EDGE_CURVE('',#11223,#11221,#5866,.T.);
#13828=EDGE_CURVE('',#11224,#11223,#6934,.T.);
#13829=EDGE_CURVE('',#11222,#11224,#5867,.T.);
#13830=EDGE_CURVE('',#11225,#11132,#6935,.T.);
#13831=EDGE_CURVE('',#11133,#11226,#6936,.T.);
#13832=EDGE_CURVE('',#11226,#11225,#6937,.T.);
#13833=EDGE_CURVE('',#11227,#11134,#6938,.T.);
#13834=EDGE_CURVE('',#11225,#11227,#5868,.T.);
#13835=EDGE_CURVE('',#11228,#11135,#6939,.T.);
#13836=EDGE_CURVE('',#11227,#11228,#6940,.T.);
#13837=EDGE_CURVE('',#11228,#11226,#5869,.T.);
#13838=EDGE_CURVE('',#11229,#11225,#6941,.T.);
#13839=EDGE_CURVE('',#11230,#11229,#5870,.T.);
#13840=EDGE_CURVE('',#11230,#11227,#6942,.T.);
#13841=EDGE_CURVE('',#11231,#11226,#6943,.T.);
#13842=EDGE_CURVE('',#11229,#11231,#6944,.T.);
#13843=EDGE_CURVE('',#11232,#11217,#6945,.T.);
#13844=EDGE_CURVE('',#11218,#11233,#6946,.T.);
#13845=EDGE_CURVE('',#11233,#11232,#6947,.T.);
#13846=EDGE_CURVE('',#11234,#11219,#6948,.T.);
#13847=EDGE_CURVE('',#11232,#11234,#5871,.T.);
#13848=EDGE_CURVE('',#11235,#11220,#6949,.T.);
#13849=EDGE_CURVE('',#11234,#11235,#6950,.T.);
#13850=EDGE_CURVE('',#11235,#11233,#5872,.T.);
#13851=EDGE_CURVE('',#11236,#11232,#6951,.T.);
#13852=EDGE_CURVE('',#11237,#11236,#5873,.T.);
#13853=EDGE_CURVE('',#11237,#11234,#6952,.T.);
#13854=EDGE_CURVE('',#11238,#11233,#6953,.T.);
#13855=EDGE_CURVE('',#11236,#11238,#6954,.T.);
#13856=EDGE_CURVE('',#11239,#11221,#6955,.T.);
#13857=EDGE_CURVE('',#11222,#11240,#6956,.T.);
#13858=EDGE_CURVE('',#11240,#11239,#6957,.T.);
#13859=EDGE_CURVE('',#11241,#11223,#6958,.T.);
#13860=EDGE_CURVE('',#11239,#11241,#5874,.T.);
#13861=EDGE_CURVE('',#11242,#11224,#6959,.T.);
#13862=EDGE_CURVE('',#11241,#11242,#6960,.T.);
#13863=EDGE_CURVE('',#11242,#11240,#5875,.T.);
#13864=EDGE_CURVE('',#11243,#11239,#6961,.T.);
#13865=EDGE_CURVE('',#11244,#11243,#5876,.T.);
#13866=EDGE_CURVE('',#11244,#11241,#6962,.T.);
#13867=EDGE_CURVE('',#11245,#11240,#6963,.T.);
#13868=EDGE_CURVE('',#11243,#11245,#6964,.T.);
#13869=EDGE_CURVE('',#11246,#11128,#6965,.T.);
#13870=EDGE_CURVE('',#11129,#11247,#6966,.T.);
#13871=EDGE_CURVE('',#11247,#11246,#6967,.T.);
#13872=EDGE_CURVE('',#11248,#11130,#6968,.T.);
#13873=EDGE_CURVE('',#11246,#11248,#5877,.T.);
#13874=EDGE_CURVE('',#11249,#11131,#6969,.T.);
#13875=EDGE_CURVE('',#11248,#11249,#6970,.T.);
#13876=EDGE_CURVE('',#11249,#11247,#5878,.T.);
#13877=EDGE_CURVE('',#11250,#11246,#6971,.T.);
#13878=EDGE_CURVE('',#11251,#11250,#5879,.T.);
#13879=EDGE_CURVE('',#11251,#11248,#6972,.T.);
#13880=EDGE_CURVE('',#11252,#11247,#6973,.T.);
#13881=EDGE_CURVE('',#11250,#11252,#6974,.T.);
#13882=EDGE_CURVE('',#11106,#11253,#5880,.T.);
#13883=EDGE_CURVE('',#11253,#11254,#6975,.T.);
#13884=EDGE_CURVE('',#11254,#11255,#5881,.T.);
#13885=EDGE_CURVE('',#11255,#11254,#5882,.T.);
#13886=EDGE_CURVE('',#11253,#11107,#5883,.T.);
#13887=EDGE_CURVE('',#11256,#11256,#5884,.T.);
#13888=EDGE_CURVE('',#11256,#11255,#6976,.T.);
#13889=EDGE_CURVE('',#11108,#11257,#5885,.T.);
#13890=EDGE_CURVE('',#11257,#11258,#6977,.T.);
#13891=EDGE_CURVE('',#11258,#11258,#5886,.T.);
#13892=EDGE_CURVE('',#11257,#11109,#5887,.T.);
#13893=EDGE_CURVE('',#11259,#11259,#5888,.T.);
#13894=EDGE_CURVE('',#11259,#11258,#6978,.T.);
#13895=EDGE_CURVE('',#11252,#11260,#6979,.T.);
#13896=EDGE_CURVE('',#11260,#11261,#6980,.T.);
#13897=EDGE_CURVE('',#11261,#11250,#6981,.T.);
#13898=EDGE_CURVE('',#11262,#11263,#6982,.T.);
#13899=EDGE_CURVE('',#11263,#11260,#5889,.T.);
#13900=EDGE_CURVE('',#11252,#11262,#5890,.T.);
#13901=EDGE_CURVE('',#11251,#11264,#6983,.T.);
#13902=EDGE_CURVE('',#11264,#11263,#6984,.T.);
#13903=EDGE_CURVE('',#11262,#11251,#6985,.T.);
#13904=EDGE_CURVE('',#11261,#11264,#5891,.T.);
#13905=EDGE_CURVE('',#11262,#11249,#6986,.T.);
#13906=EDGE_CURVE('',#11265,#11266,#205,.T.);
#13907=EDGE_CURVE('',#11267,#11265,#6987,.T.);
#13908=EDGE_CURVE('',#11268,#11267,#6988,.T.);
#13909=EDGE_CURVE('',#11269,#11268,#6989,.F.);
#13910=EDGE_CURVE('',#11270,#11269,#6990,.T.);
#13911=EDGE_CURVE('',#11271,#11270,#6991,.F.);
#13912=EDGE_CURVE('',#11271,#11272,#6992,.T.);
#13913=EDGE_CURVE('',#11273,#11272,#6993,.T.);
#13914=EDGE_CURVE('',#11161,#11273,#6994,.T.);
#13915=EDGE_CURVE('',#11274,#11163,#6995,.F.);
#13916=EDGE_CURVE('',#11274,#11275,#6996,.T.);
#13917=EDGE_CURVE('',#11276,#11275,#6997,.T.);
#13918=EDGE_CURVE('',#11277,#11276,#206,.T.);
#13919=EDGE_CURVE('',#11278,#11277,#5892,.T.);
#13920=EDGE_CURVE('',#11279,#11278,#6998,.T.);
#13921=EDGE_CURVE('',#11280,#11279,#5893,.T.);
#13922=EDGE_CURVE('',#11281,#11280,#6999,.T.);
#13923=EDGE_CURVE('',#11282,#11281,#5894,.T.);
#13924=EDGE_CURVE('',#11283,#11282,#7000,.T.);
#13925=EDGE_CURVE('',#11266,#11283,#5895,.T.);
#13926=EDGE_CURVE('',#11284,#11285,#7001,.T.);
#13927=EDGE_CURVE('',#11286,#11284,#5896,.T.);
#13928=EDGE_CURVE('',#11287,#11286,#7002,.T.);
#13929=EDGE_CURVE('',#11285,#11287,#5897,.T.);
#13930=EDGE_CURVE('',#11288,#11289,#7003,.T.);
#13931=EDGE_CURVE('',#11290,#11288,#5898,.T.);
#13932=EDGE_CURVE('',#11291,#11290,#7004,.T.);
#13933=EDGE_CURVE('',#11289,#11291,#5899,.T.);
#13934=EDGE_CURVE('',#11292,#11293,#7005,.T.);
#13935=EDGE_CURVE('',#11294,#11292,#5900,.T.);
#13936=EDGE_CURVE('',#11295,#11294,#7006,.T.);
#13937=EDGE_CURVE('',#11293,#11295,#5901,.T.);
#13938=EDGE_CURVE('',#11245,#11284,#7007,.T.);
#13939=EDGE_CURVE('',#11285,#11243,#7008,.T.);
#13940=EDGE_CURVE('',#11296,#11286,#7009,.T.);
#13941=EDGE_CURVE('',#11245,#11296,#5902,.T.);
#13942=EDGE_CURVE('',#11244,#11287,#7010,.T.);
#13943=EDGE_CURVE('',#11296,#11244,#7011,.T.);
#13944=EDGE_CURVE('',#11296,#11242,#7012,.T.);
#13945=EDGE_CURVE('',#11238,#11292,#7013,.T.);
#13946=EDGE_CURVE('',#11293,#11236,#7014,.T.);
#13947=EDGE_CURVE('',#11297,#11294,#7015,.T.);
#13948=EDGE_CURVE('',#11238,#11297,#5903,.T.);
#13949=EDGE_CURVE('',#11237,#11295,#7016,.T.);
#13950=EDGE_CURVE('',#11297,#11237,#7017,.T.);
#13951=EDGE_CURVE('',#11297,#11235,#7018,.T.);
#13952=EDGE_CURVE('',#11231,#11288,#7019,.T.);
#13953=EDGE_CURVE('',#11289,#11229,#7020,.T.);
#13954=EDGE_CURVE('',#11298,#11290,#7021,.T.);
#13955=EDGE_CURVE('',#11231,#11298,#5904,.T.);
#13956=EDGE_CURVE('',#11230,#11291,#7022,.T.);
#13957=EDGE_CURVE('',#11298,#11230,#7023,.T.);
#13958=EDGE_CURVE('',#11298,#11228,#7024,.T.);
#13959=EDGE_CURVE('',#11212,#11299,#207,.T.);
#13960=EDGE_CURVE('',#11203,#11299,#208,.T.);
#13961=EDGE_CURVE('',#11206,#11300,#209,.T.);
#13962=EDGE_CURVE('',#11301,#11300,#210,.T.);
#13963=EDGE_CURVE('',#11301,#11207,#211,.T.);
#13964=EDGE_CURVE('',#11300,#11302,#212,.T.);
#13965=EDGE_CURVE('',#11302,#11276,#7025,.T.);
#13966=EDGE_CURVE('',#11276,#11301,#213,.T.);
#13967=EDGE_CURVE('',#11303,#11278,#7026,.T.);
#13968=EDGE_CURVE('',#11277,#11304,#7027,.T.);
#13969=EDGE_CURVE('',#11304,#11303,#5905,.T.);
#13970=EDGE_CURVE('',#11305,#11279,#7028,.T.);
#13971=EDGE_CURVE('',#11303,#11305,#7029,.T.);
#13972=EDGE_CURVE('',#11306,#11280,#7030,.T.);
#13973=EDGE_CURVE('',#11305,#11306,#5906,.T.);
#13974=EDGE_CURVE('',#11307,#11281,#7031,.T.);
#13975=EDGE_CURVE('',#11306,#11307,#7032,.T.);
#13976=EDGE_CURVE('',#11201,#11282,#7033,.T.);
#13977=EDGE_CURVE('',#11307,#11201,#5907,.T.);
#13978=EDGE_CURVE('',#11200,#11283,#7034,.T.);
#13979=EDGE_CURVE('',#11205,#11266,#7035,.T.);
#13980=EDGE_CURVE('',#11302,#11304,#214,.T.);
#13981=EDGE_CURVE('',#11299,#11265,#215,.T.);
#13982=EDGE_CURVE('',#11265,#11204,#7036,.T.);
#13983=EDGE_CURVE('',#11267,#11211,#1093,.F.);
#13984=EDGE_CURVE('',#11192,#11307,#7037,.T.);
#13985=EDGE_CURVE('',#11190,#11306,#7038,.T.);
#13986=EDGE_CURVE('',#11188,#11305,#7039,.T.);
#13987=EDGE_CURVE('',#11137,#11303,#7040,.T.);
#13988=EDGE_CURVE('',#11308,#11271,#7041,.T.);
#13989=EDGE_CURVE('',#11270,#11309,#7042,.T.);
#13990=EDGE_CURVE('',#11309,#11308,#216,.T.);
#13991=EDGE_CURVE('',#11309,#11310,#5908,.T.);
#13992=EDGE_CURVE('',#11310,#11311,#7043,.T.);
#13993=EDGE_CURVE('',#11311,#11308,#5909,.T.);
#13994=EDGE_CURVE('',#11312,#11313,#7044,.T.);
#13995=EDGE_CURVE('',#11313,#11314,#217,.T.);
#13996=EDGE_CURVE('',#11314,#11315,#7045,.T.);
#13997=EDGE_CURVE('',#11315,#11312,#218,.T.);
#13998=EDGE_CURVE('',#11312,#11311,#219,.T.);
#13999=EDGE_CURVE('',#11310,#11313,#220,.T.);
#14000=EDGE_CURVE('',#11164,#11315,#221,.T.);
#14001=EDGE_CURVE('',#11314,#11165,#222,.T.);
#14002=EDGE_CURVE('',#11312,#11316,#7046,.T.);
#14003=EDGE_CURVE('',#11272,#11316,#7047,.T.);
#14004=EDGE_CURVE('',#11315,#11317,#7048,.T.);
#14005=EDGE_CURVE('',#11316,#11317,#5910,.T.);
#14006=EDGE_CURVE('',#11317,#11273,#7049,.T.);
#14007=EDGE_CURVE('',#11318,#11269,#7050,.T.);
#14008=EDGE_CURVE('',#11268,#11319,#7051,.T.);
#14009=EDGE_CURVE('',#11319,#11320,#223,.T.);
#14010=EDGE_CURVE('',#11320,#11318,#1094,.T.);
#14011=EDGE_CURVE('',#11319,#11153,#224,.T.);
#14012=EDGE_CURVE('',#11152,#11320,#225,.T.);
#14013=EDGE_CURVE('',#11318,#11309,#7052,.T.);
#14014=EDGE_CURVE('',#11321,#11151,#226,.T.);
#14015=EDGE_CURVE('',#11162,#11321,#1095,.T.);
#14016=EDGE_CURVE('',#11322,#11274,#7053,.T.);
#14017=EDGE_CURVE('',#11321,#11322,#227,.T.);
#14018=EDGE_CURVE('',#11150,#11322,#228,.T.);
#14019=EDGE_CURVE('',#11323,#11149,#229,.T.);
#14020=EDGE_CURVE('',#11275,#11323,#7054,.T.);
#14021=EDGE_CURVE('',#11323,#11209,#5911,.T.);
#14022=EDGE_CURVE('',#11208,#11275,#1096,.F.);
#14023=EDGE_CURVE('',#11156,#11209,#230,.T.);
#14024=EDGE_CURVE('',#11324,#11210,#5912,.T.);
#14025=EDGE_CURVE('',#11210,#11155,#231,.T.);
#14026=EDGE_CURVE('',#11154,#11324,#232,.T.);
#14027=EDGE_CURVE('',#11324,#11267,#7055,.T.);
#14028=EDGE_CURVE('',#11316,#11213,#5913,.T.);
#14029=EDGE_CURVE('',#11214,#11272,#1097,.T.);
#14030=EDGE_CURVE('',#11216,#11273,#1098,.T.);
#14031=EDGE_CURVE('',#11317,#11215,#5914,.T.);
#14032=EDGE_CURVE('',#11325,#11115,#7056,.T.);
#14033=EDGE_CURVE('',#11326,#11259,#7057,.T.);
#14034=EDGE_CURVE('',#11327,#11256,#7058,.T.);
#14035=EDGE_CURVE('',#11328,#11112,#7059,.T.);
#14036=EDGE_CURVE('',#11329,#11329,#5915,.T.);
#14037=EDGE_CURVE('',#11329,#11330,#7060,.T.);
#14038=EDGE_CURVE('',#11331,#11330,#233,.T.);
#14039=EDGE_CURVE('',#11330,#11331,#234,.T.);
#14040=EDGE_CURVE('',#11332,#11333,#235,.T.);
#14041=EDGE_CURVE('',#11333,#11332,#236,.T.);
#14042=EDGE_CURVE('',#11333,#11334,#7061,.T.);
#14043=EDGE_CURVE('',#11334,#11334,#5916,.T.);
#14044=EDGE_CURVE('',#11335,#11335,#5917,.T.);
#14045=EDGE_CURVE('',#11335,#11093,#7062,.T.);
#14046=EDGE_CURVE('',#11336,#11336,#5918,.T.);
#14047=EDGE_CURVE('',#11336,#11143,#7063,.T.);
#17837=ORIENTED_EDGE('',*,*,#13641,.T.);
#17838=ORIENTED_EDGE('',*,*,#13642,.T.);
#17839=ORIENTED_EDGE('',*,*,#13643,.T.);
#17840=ORIENTED_EDGE('',*,*,#13644,.T.);
#17841=ORIENTED_EDGE('',*,*,#13642,.F.);
#17842=ORIENTED_EDGE('',*,*,#13643,.F.);
#17843=ORIENTED_EDGE('',*,*,#13644,.F.);
#17844=ORIENTED_EDGE('',*,*,#13645,.T.);
#17845=ORIENTED_EDGE('',*,*,#13646,.F.);
#17846=ORIENTED_EDGE('',*,*,#13647,.F.);
#17847=ORIENTED_EDGE('',*,*,#13645,.F.);
#17848=ORIENTED_EDGE('',*,*,#13641,.F.);
#17849=ORIENTED_EDGE('',*,*,#13648,.T.);
#17850=ORIENTED_EDGE('',*,*,#13646,.T.);
#17851=ORIENTED_EDGE('',*,*,#13647,.T.);
#17852=ORIENTED_EDGE('',*,*,#13649,.T.);
#17853=ORIENTED_EDGE('',*,*,#13650,.T.);
#17854=ORIENTED_EDGE('',*,*,#13651,.T.);
#17855=ORIENTED_EDGE('',*,*,#13649,.F.);
#17856=ORIENTED_EDGE('',*,*,#13650,.F.);
#17857=ORIENTED_EDGE('',*,*,#13651,.F.);
#17858=ORIENTED_EDGE('',*,*,#13652,.T.);
#17859=ORIENTED_EDGE('',*,*,#13653,.F.);
#17860=ORIENTED_EDGE('',*,*,#13654,.F.);
#17861=ORIENTED_EDGE('',*,*,#13652,.F.);
#17862=ORIENTED_EDGE('',*,*,#13655,.T.);
#17863=ORIENTED_EDGE('',*,*,#13656,.T.);
#17864=ORIENTED_EDGE('',*,*,#13657,.T.);
#17865=ORIENTED_EDGE('',*,*,#13658,.T.);
#17866=ORIENTED_EDGE('',*,*,#13659,.T.);
#17867=ORIENTED_EDGE('',*,*,#13657,.F.);
#17868=ORIENTED_EDGE('',*,*,#13660,.T.);
#17869=ORIENTED_EDGE('',*,*,#13661,.T.);
#17870=ORIENTED_EDGE('',*,*,#13662,.T.);
#17871=ORIENTED_EDGE('',*,*,#13663,.T.);
#17872=ORIENTED_EDGE('',*,*,#13664,.T.);
#17873=ORIENTED_EDGE('',*,*,#13655,.F.);
#17874=ORIENTED_EDGE('',*,*,#13665,.T.);
#17875=ORIENTED_EDGE('',*,*,#13666,.F.);
#17876=ORIENTED_EDGE('',*,*,#13667,.T.);
#17877=ORIENTED_EDGE('',*,*,#13668,.F.);
#17878=ORIENTED_EDGE('',*,*,#13669,.T.);
#17879=ORIENTED_EDGE('',*,*,#13670,.F.);
#17880=ORIENTED_EDGE('',*,*,#13671,.T.);
#17881=ORIENTED_EDGE('',*,*,#13663,.F.);
#17882=ORIENTED_EDGE('',*,*,#13672,.F.);
#17883=ORIENTED_EDGE('',*,*,#13673,.T.);
#17884=ORIENTED_EDGE('',*,*,#13658,.F.);
#17885=ORIENTED_EDGE('',*,*,#13659,.F.);
#17886=ORIENTED_EDGE('',*,*,#13673,.F.);
#17887=ORIENTED_EDGE('',*,*,#13670,.T.);
#17888=ORIENTED_EDGE('',*,*,#13674,.T.);
#17889=ORIENTED_EDGE('',*,*,#13675,.T.);
#17890=ORIENTED_EDGE('',*,*,#13676,.T.);
#17891=ORIENTED_EDGE('',*,*,#13675,.F.);
#17892=ORIENTED_EDGE('',*,*,#13677,.T.);
#17893=ORIENTED_EDGE('',*,*,#13678,.F.);
#17894=ORIENTED_EDGE('',*,*,#13679,.T.);
#17895=ORIENTED_EDGE('',*,*,#13676,.F.);
#17896=ORIENTED_EDGE('',*,*,#13679,.F.);
#17897=ORIENTED_EDGE('',*,*,#13680,.T.);
#17898=ORIENTED_EDGE('',*,*,#13681,.T.);
#17899=ORIENTED_EDGE('',*,*,#13682,.T.);
#17900=ORIENTED_EDGE('',*,*,#13683,.T.);
#17901=ORIENTED_EDGE('',*,*,#13684,.T.);
#17902=ORIENTED_EDGE('',*,*,#13685,.T.);
#17903=ORIENTED_EDGE('',*,*,#13681,.F.);
#17904=ORIENTED_EDGE('',*,*,#13686,.F.);
#17905=ORIENTED_EDGE('',*,*,#13687,.F.);
#17906=ORIENTED_EDGE('',*,*,#13688,.F.);
#17907=ORIENTED_EDGE('',*,*,#13689,.F.);
#17908=ORIENTED_EDGE('',*,*,#13690,.F.);
#17909=ORIENTED_EDGE('',*,*,#13691,.F.);
#17910=ORIENTED_EDGE('',*,*,#13692,.F.);
#17911=ORIENTED_EDGE('',*,*,#13693,.F.);
#17912=ORIENTED_EDGE('',*,*,#13694,.F.);
#17913=ORIENTED_EDGE('',*,*,#13695,.F.);
#17914=ORIENTED_EDGE('',*,*,#13696,.F.);
#17915=ORIENTED_EDGE('',*,*,#13697,.F.);
#17916=ORIENTED_EDGE('',*,*,#13698,.F.);
#17917=ORIENTED_EDGE('',*,*,#13699,.F.);
#17918=ORIENTED_EDGE('',*,*,#13700,.F.);
#17919=ORIENTED_EDGE('',*,*,#13680,.F.);
#17920=ORIENTED_EDGE('',*,*,#13701,.F.);
#17921=ORIENTED_EDGE('',*,*,#13702,.T.);
#17922=ORIENTED_EDGE('',*,*,#13703,.T.);
#17923=ORIENTED_EDGE('',*,*,#13686,.T.);
#17924=ORIENTED_EDGE('',*,*,#13685,.F.);
#17925=ORIENTED_EDGE('',*,*,#13704,.T.);
#17926=ORIENTED_EDGE('',*,*,#13705,.T.);
#17927=ORIENTED_EDGE('',*,*,#13706,.T.);
#17928=ORIENTED_EDGE('',*,*,#13701,.T.);
#17929=ORIENTED_EDGE('',*,*,#13707,.T.);
#17930=ORIENTED_EDGE('',*,*,#13708,.T.);
#17931=ORIENTED_EDGE('',*,*,#13709,.T.);
#17932=ORIENTED_EDGE('',*,*,#13708,.F.);
#17933=ORIENTED_EDGE('',*,*,#13707,.F.);
#17934=ORIENTED_EDGE('',*,*,#13710,.T.);
#17935=ORIENTED_EDGE('',*,*,#13711,.F.);
#17936=ORIENTED_EDGE('',*,*,#13710,.F.);
#17937=ORIENTED_EDGE('',*,*,#13709,.F.);
#17938=ORIENTED_EDGE('',*,*,#13712,.T.);
#17939=ORIENTED_EDGE('',*,*,#13713,.T.);
#17940=ORIENTED_EDGE('',*,*,#13714,.T.);
#17941=ORIENTED_EDGE('',*,*,#13715,.T.);
#17942=ORIENTED_EDGE('',*,*,#13713,.F.);
#17943=ORIENTED_EDGE('',*,*,#13716,.T.);
#17944=ORIENTED_EDGE('',*,*,#13717,.F.);
#17945=ORIENTED_EDGE('',*,*,#13718,.F.);
#17946=ORIENTED_EDGE('',*,*,#13719,.T.);
#17947=ORIENTED_EDGE('',*,*,#13661,.F.);
#17948=ORIENTED_EDGE('',*,*,#13662,.F.);
#17949=ORIENTED_EDGE('',*,*,#13719,.F.);
#17950=ORIENTED_EDGE('',*,*,#13720,.T.);
#17951=ORIENTED_EDGE('',*,*,#13721,.F.);
#17952=ORIENTED_EDGE('',*,*,#13722,.T.);
#17953=ORIENTED_EDGE('',*,*,#13723,.F.);
#17954=ORIENTED_EDGE('',*,*,#13724,.T.);
#17955=ORIENTED_EDGE('',*,*,#13725,.F.);
#17956=ORIENTED_EDGE('',*,*,#13726,.F.);
#17957=ORIENTED_EDGE('',*,*,#13727,.F.);
#17958=ORIENTED_EDGE('',*,*,#13653,.T.);
#17959=ORIENTED_EDGE('',*,*,#13654,.T.);
#17960=ORIENTED_EDGE('',*,*,#13716,.F.);
#17961=ORIENTED_EDGE('',*,*,#13714,.F.);
#17962=ORIENTED_EDGE('',*,*,#13715,.F.);
#17963=ORIENTED_EDGE('',*,*,#13728,.T.);
#17964=ORIENTED_EDGE('',*,*,#13729,.T.);
#17965=ORIENTED_EDGE('',*,*,#13728,.F.);
#17966=ORIENTED_EDGE('',*,*,#13711,.T.);
#17967=ORIENTED_EDGE('',*,*,#13730,.T.);
#17968=ORIENTED_EDGE('',*,*,#13717,.T.);
#17969=ORIENTED_EDGE('',*,*,#13718,.T.);
#17970=ORIENTED_EDGE('',*,*,#13730,.F.);
#17971=ORIENTED_EDGE('',*,*,#13731,.T.);
#17972=ORIENTED_EDGE('',*,*,#13732,.T.);
#17973=ORIENTED_EDGE('',*,*,#13733,.T.);
#17974=ORIENTED_EDGE('',*,*,#13734,.T.);
#17975=ORIENTED_EDGE('',*,*,#13732,.F.);
#17976=ORIENTED_EDGE('',*,*,#13735,.T.);
#17977=ORIENTED_EDGE('',*,*,#13736,.F.);
#17978=ORIENTED_EDGE('',*,*,#13737,.T.);
#17979=ORIENTED_EDGE('',*,*,#13731,.F.);
#17980=ORIENTED_EDGE('',*,*,#13738,.T.);
#17981=ORIENTED_EDGE('',*,*,#13739,.T.);
#17982=ORIENTED_EDGE('',*,*,#13740,.T.);
#17983=ORIENTED_EDGE('',*,*,#13741,.T.);
#17984=ORIENTED_EDGE('',*,*,#13742,.F.);
#17985=ORIENTED_EDGE('',*,*,#13743,.T.);
#17986=ORIENTED_EDGE('',*,*,#13744,.T.);
#17987=ORIENTED_EDGE('',*,*,#13745,.T.);
#17988=ORIENTED_EDGE('',*,*,#13746,.F.);
#17989=ORIENTED_EDGE('',*,*,#13747,.T.);
#17990=ORIENTED_EDGE('',*,*,#13748,.T.);
#17991=ORIENTED_EDGE('',*,*,#13746,.T.);
#17992=ORIENTED_EDGE('',*,*,#13749,.T.);
#17993=ORIENTED_EDGE('',*,*,#13750,.T.);
#17994=ORIENTED_EDGE('',*,*,#13751,.T.);
#17995=ORIENTED_EDGE('',*,*,#13682,.F.);
#17996=ORIENTED_EDGE('',*,*,#13692,.T.);
#17997=ORIENTED_EDGE('',*,*,#13752,.T.);
#17998=ORIENTED_EDGE('',*,*,#13753,.T.);
#17999=ORIENTED_EDGE('',*,*,#13754,.T.);
#18000=ORIENTED_EDGE('',*,*,#13683,.F.);
#18001=ORIENTED_EDGE('',*,*,#13754,.F.);
#18002=ORIENTED_EDGE('',*,*,#13755,.T.);
#18003=ORIENTED_EDGE('',*,*,#13756,.T.);
#18004=ORIENTED_EDGE('',*,*,#13757,.T.);
#18005=ORIENTED_EDGE('',*,*,#13758,.F.);
#18006=ORIENTED_EDGE('',*,*,#13759,.F.);
#18007=ORIENTED_EDGE('',*,*,#13760,.F.);
#18008=ORIENTED_EDGE('',*,*,#13761,.T.);
#18009=ORIENTED_EDGE('',*,*,#13759,.T.);
#18010=ORIENTED_EDGE('',*,*,#13762,.T.);
#18011=ORIENTED_EDGE('',*,*,#13763,.T.);
#18012=ORIENTED_EDGE('',*,*,#13764,.F.);
#18013=ORIENTED_EDGE('',*,*,#13765,.F.);
#18014=ORIENTED_EDGE('',*,*,#13766,.F.);
#18015=ORIENTED_EDGE('',*,*,#13767,.T.);
#18016=ORIENTED_EDGE('',*,*,#13768,.T.);
#18017=ORIENTED_EDGE('',*,*,#13765,.T.);
#18018=ORIENTED_EDGE('',*,*,#13769,.T.);
#18019=ORIENTED_EDGE('',*,*,#13770,.T.);
#18020=ORIENTED_EDGE('',*,*,#13771,.T.);
#18021=ORIENTED_EDGE('',*,*,#13767,.F.);
#18022=ORIENTED_EDGE('',*,*,#13772,.T.);
#18023=ORIENTED_EDGE('',*,*,#13773,.T.);
#18024=ORIENTED_EDGE('',*,*,#13774,.T.);
#18025=ORIENTED_EDGE('',*,*,#13770,.F.);
#18026=ORIENTED_EDGE('',*,*,#13775,.T.);
#18027=ORIENTED_EDGE('',*,*,#13776,.T.);
#18028=ORIENTED_EDGE('',*,*,#13777,.T.);
#18029=ORIENTED_EDGE('',*,*,#13773,.F.);
#18030=ORIENTED_EDGE('',*,*,#13778,.T.);
#18031=ORIENTED_EDGE('',*,*,#13776,.F.);
#18032=ORIENTED_EDGE('',*,*,#13779,.T.);
#18033=ORIENTED_EDGE('',*,*,#13760,.T.);
#18034=ORIENTED_EDGE('',*,*,#13780,.T.);
#18035=ORIENTED_EDGE('',*,*,#13781,.T.);
#18036=ORIENTED_EDGE('',*,*,#13766,.T.);
#18037=ORIENTED_EDGE('',*,*,#13782,.T.);
#18038=ORIENTED_EDGE('',*,*,#13783,.T.);
#18039=ORIENTED_EDGE('',*,*,#13758,.T.);
#18040=ORIENTED_EDGE('',*,*,#13784,.T.);
#18041=ORIENTED_EDGE('',*,*,#13764,.T.);
#18042=ORIENTED_EDGE('',*,*,#13785,.T.);
#18043=ORIENTED_EDGE('',*,*,#13786,.T.);
#18044=ORIENTED_EDGE('',*,*,#13783,.F.);
#18045=ORIENTED_EDGE('',*,*,#13787,.T.);
#18046=ORIENTED_EDGE('',*,*,#13705,.F.);
#18047=ORIENTED_EDGE('',*,*,#13788,.T.);
#18048=ORIENTED_EDGE('',*,*,#13763,.F.);
#18049=ORIENTED_EDGE('',*,*,#13789,.T.);
#18050=ORIENTED_EDGE('',*,*,#13756,.F.);
#18051=ORIENTED_EDGE('',*,*,#13703,.F.);
#18052=ORIENTED_EDGE('',*,*,#13790,.T.);
#18053=ORIENTED_EDGE('',*,*,#13791,.T.);
#18054=ORIENTED_EDGE('',*,*,#13687,.T.);
#18055=ORIENTED_EDGE('',*,*,#13792,.T.);
#18056=ORIENTED_EDGE('',*,*,#13793,.T.);
#18057=ORIENTED_EDGE('',*,*,#13752,.F.);
#18058=ORIENTED_EDGE('',*,*,#13691,.T.);
#18059=ORIENTED_EDGE('',*,*,#13791,.F.);
#18060=ORIENTED_EDGE('',*,*,#13794,.T.);
#18061=ORIENTED_EDGE('',*,*,#13750,.F.);
#18062=ORIENTED_EDGE('',*,*,#13688,.T.);
#18063=ORIENTED_EDGE('',*,*,#13742,.T.);
#18064=ORIENTED_EDGE('',*,*,#13795,.T.);
#18065=ORIENTED_EDGE('',*,*,#13796,.T.);
#18066=ORIENTED_EDGE('',*,*,#13797,.T.);
#18067=ORIENTED_EDGE('',*,*,#13796,.F.);
#18068=ORIENTED_EDGE('',*,*,#13798,.T.);
#18069=ORIENTED_EDGE('',*,*,#13792,.F.);
#18070=ORIENTED_EDGE('',*,*,#13690,.T.);
#18071=ORIENTED_EDGE('',*,*,#13780,.F.);
#18072=ORIENTED_EDGE('',*,*,#13761,.F.);
#18073=ORIENTED_EDGE('',*,*,#13788,.F.);
#18074=ORIENTED_EDGE('',*,*,#13755,.F.);
#18075=ORIENTED_EDGE('',*,*,#13753,.F.);
#18076=ORIENTED_EDGE('',*,*,#13799,.T.);
#18077=ORIENTED_EDGE('',*,*,#13800,.F.);
#18078=ORIENTED_EDGE('',*,*,#13801,.F.);
#18079=ORIENTED_EDGE('',*,*,#13793,.F.);
#18080=ORIENTED_EDGE('',*,*,#13798,.F.);
#18081=ORIENTED_EDGE('',*,*,#13795,.F.);
#18082=ORIENTED_EDGE('',*,*,#13741,.F.);
#18083=ORIENTED_EDGE('',*,*,#13802,.T.);
#18084=ORIENTED_EDGE('',*,*,#13803,.F.);
#18085=ORIENTED_EDGE('',*,*,#13804,.F.);
#18086=ORIENTED_EDGE('',*,*,#13805,.F.);
#18087=ORIENTED_EDGE('',*,*,#13806,.F.);
#18088=ORIENTED_EDGE('',*,*,#13799,.F.);
#18089=ORIENTED_EDGE('',*,*,#13744,.F.);
#18090=ORIENTED_EDGE('',*,*,#13807,.F.);
#18091=ORIENTED_EDGE('',*,*,#13748,.F.);
#18092=ORIENTED_EDGE('',*,*,#13808,.T.);
#18093=ORIENTED_EDGE('',*,*,#13809,.F.);
#18094=ORIENTED_EDGE('',*,*,#13810,.F.);
#18095=ORIENTED_EDGE('',*,*,#13811,.F.);
#18096=ORIENTED_EDGE('',*,*,#13812,.F.);
#18097=ORIENTED_EDGE('',*,*,#13813,.F.);
#18098=ORIENTED_EDGE('',*,*,#13814,.F.);
#18099=ORIENTED_EDGE('',*,*,#13815,.F.);
#18100=ORIENTED_EDGE('',*,*,#13802,.F.);
#18101=ORIENTED_EDGE('',*,*,#13816,.F.);
#18102=ORIENTED_EDGE('',*,*,#13817,.F.);
#18103=ORIENTED_EDGE('',*,*,#13818,.F.);
#18104=ORIENTED_EDGE('',*,*,#13819,.F.);
#18105=ORIENTED_EDGE('',*,*,#13743,.F.);
#18106=ORIENTED_EDGE('',*,*,#13797,.F.);
#18107=ORIENTED_EDGE('',*,*,#13689,.T.);
#18108=ORIENTED_EDGE('',*,*,#13749,.F.);
#18109=ORIENTED_EDGE('',*,*,#13745,.F.);
#18110=ORIENTED_EDGE('',*,*,#13807,.T.);
#18111=ORIENTED_EDGE('',*,*,#13762,.F.);
#18112=ORIENTED_EDGE('',*,*,#13785,.F.);
#18113=ORIENTED_EDGE('',*,*,#13781,.F.);
#18114=ORIENTED_EDGE('',*,*,#13820,.T.);
#18115=ORIENTED_EDGE('',*,*,#13684,.F.);
#18116=ORIENTED_EDGE('',*,*,#13757,.F.);
#18117=ORIENTED_EDGE('',*,*,#13821,.T.);
#18118=ORIENTED_EDGE('',*,*,#13704,.F.);
#18119=ORIENTED_EDGE('',*,*,#13789,.F.);
#18120=ORIENTED_EDGE('',*,*,#13820,.F.);
#18121=ORIENTED_EDGE('',*,*,#13786,.F.);
#18122=ORIENTED_EDGE('',*,*,#13821,.F.);
#18123=ORIENTED_EDGE('',*,*,#13769,.F.);
#18124=ORIENTED_EDGE('',*,*,#13784,.F.);
#18125=ORIENTED_EDGE('',*,*,#13779,.F.);
#18126=ORIENTED_EDGE('',*,*,#13778,.F.);
#18127=ORIENTED_EDGE('',*,*,#13775,.F.);
#18128=ORIENTED_EDGE('',*,*,#13772,.F.);
#18129=ORIENTED_EDGE('',*,*,#13822,.F.);
#18130=ORIENTED_EDGE('',*,*,#13823,.F.);
#18131=ORIENTED_EDGE('',*,*,#13824,.F.);
#18132=ORIENTED_EDGE('',*,*,#13825,.F.);
#18133=ORIENTED_EDGE('',*,*,#13826,.F.);
#18134=ORIENTED_EDGE('',*,*,#13827,.F.);
#18135=ORIENTED_EDGE('',*,*,#13828,.F.);
#18136=ORIENTED_EDGE('',*,*,#13829,.F.);
#18137=ORIENTED_EDGE('',*,*,#13830,.T.);
#18138=ORIENTED_EDGE('',*,*,#13697,.T.);
#18139=ORIENTED_EDGE('',*,*,#13831,.T.);
#18140=ORIENTED_EDGE('',*,*,#13832,.T.);
#18141=ORIENTED_EDGE('',*,*,#13833,.T.);
#18142=ORIENTED_EDGE('',*,*,#13698,.T.);
#18143=ORIENTED_EDGE('',*,*,#13830,.F.);
#18144=ORIENTED_EDGE('',*,*,#13834,.T.);
#18145=ORIENTED_EDGE('',*,*,#13835,.T.);
#18146=ORIENTED_EDGE('',*,*,#13699,.T.);
#18147=ORIENTED_EDGE('',*,*,#13833,.F.);
#18148=ORIENTED_EDGE('',*,*,#13836,.T.);
#18149=ORIENTED_EDGE('',*,*,#13831,.F.);
#18150=ORIENTED_EDGE('',*,*,#13700,.T.);
#18151=ORIENTED_EDGE('',*,*,#13835,.F.);
#18152=ORIENTED_EDGE('',*,*,#13837,.T.);
#18153=ORIENTED_EDGE('',*,*,#13834,.F.);
#18154=ORIENTED_EDGE('',*,*,#13838,.F.);
#18155=ORIENTED_EDGE('',*,*,#13839,.F.);
#18156=ORIENTED_EDGE('',*,*,#13840,.T.);
#18157=ORIENTED_EDGE('',*,*,#13832,.F.);
#18158=ORIENTED_EDGE('',*,*,#13841,.F.);
#18159=ORIENTED_EDGE('',*,*,#13842,.F.);
#18160=ORIENTED_EDGE('',*,*,#13838,.T.);
#18161=ORIENTED_EDGE('',*,*,#13843,.T.);
#18162=ORIENTED_EDGE('',*,*,#13822,.T.);
#18163=ORIENTED_EDGE('',*,*,#13844,.T.);
#18164=ORIENTED_EDGE('',*,*,#13845,.T.);
#18165=ORIENTED_EDGE('',*,*,#13846,.T.);
#18166=ORIENTED_EDGE('',*,*,#13823,.T.);
#18167=ORIENTED_EDGE('',*,*,#13843,.F.);
#18168=ORIENTED_EDGE('',*,*,#13847,.T.);
#18169=ORIENTED_EDGE('',*,*,#13848,.T.);
#18170=ORIENTED_EDGE('',*,*,#13824,.T.);
#18171=ORIENTED_EDGE('',*,*,#13846,.F.);
#18172=ORIENTED_EDGE('',*,*,#13849,.T.);
#18173=ORIENTED_EDGE('',*,*,#13844,.F.);
#18174=ORIENTED_EDGE('',*,*,#13825,.T.);
#18175=ORIENTED_EDGE('',*,*,#13848,.F.);
#18176=ORIENTED_EDGE('',*,*,#13850,.T.);
#18177=ORIENTED_EDGE('',*,*,#13847,.F.);
#18178=ORIENTED_EDGE('',*,*,#13851,.F.);
#18179=ORIENTED_EDGE('',*,*,#13852,.F.);
#18180=ORIENTED_EDGE('',*,*,#13853,.T.);
#18181=ORIENTED_EDGE('',*,*,#13845,.F.);
#18182=ORIENTED_EDGE('',*,*,#13854,.F.);
#18183=ORIENTED_EDGE('',*,*,#13855,.F.);
#18184=ORIENTED_EDGE('',*,*,#13851,.T.);
#18185=ORIENTED_EDGE('',*,*,#13856,.T.);
#18186=ORIENTED_EDGE('',*,*,#13826,.T.);
#18187=ORIENTED_EDGE('',*,*,#13857,.T.);
#18188=ORIENTED_EDGE('',*,*,#13858,.T.);
#18189=ORIENTED_EDGE('',*,*,#13859,.T.);
#18190=ORIENTED_EDGE('',*,*,#13827,.T.);
#18191=ORIENTED_EDGE('',*,*,#13856,.F.);
#18192=ORIENTED_EDGE('',*,*,#13860,.T.);
#18193=ORIENTED_EDGE('',*,*,#13861,.T.);
#18194=ORIENTED_EDGE('',*,*,#13828,.T.);
#18195=ORIENTED_EDGE('',*,*,#13859,.F.);
#18196=ORIENTED_EDGE('',*,*,#13862,.T.);
#18197=ORIENTED_EDGE('',*,*,#13857,.F.);
#18198=ORIENTED_EDGE('',*,*,#13829,.T.);
#18199=ORIENTED_EDGE('',*,*,#13861,.F.);
#18200=ORIENTED_EDGE('',*,*,#13863,.T.);
#18201=ORIENTED_EDGE('',*,*,#13860,.F.);
#18202=ORIENTED_EDGE('',*,*,#13864,.F.);
#18203=ORIENTED_EDGE('',*,*,#13865,.F.);
#18204=ORIENTED_EDGE('',*,*,#13866,.T.);
#18205=ORIENTED_EDGE('',*,*,#13858,.F.);
#18206=ORIENTED_EDGE('',*,*,#13867,.F.);
#18207=ORIENTED_EDGE('',*,*,#13868,.F.);
#18208=ORIENTED_EDGE('',*,*,#13864,.T.);
#18209=ORIENTED_EDGE('',*,*,#13869,.T.);
#18210=ORIENTED_EDGE('',*,*,#13693,.T.);
#18211=ORIENTED_EDGE('',*,*,#13870,.T.);
#18212=ORIENTED_EDGE('',*,*,#13871,.T.);
#18213=ORIENTED_EDGE('',*,*,#13872,.T.);
#18214=ORIENTED_EDGE('',*,*,#13694,.T.);
#18215=ORIENTED_EDGE('',*,*,#13869,.F.);
#18216=ORIENTED_EDGE('',*,*,#13873,.T.);
#18217=ORIENTED_EDGE('',*,*,#13874,.T.);
#18218=ORIENTED_EDGE('',*,*,#13695,.T.);
#18219=ORIENTED_EDGE('',*,*,#13872,.F.);
#18220=ORIENTED_EDGE('',*,*,#13875,.T.);
#18221=ORIENTED_EDGE('',*,*,#13870,.F.);
#18222=ORIENTED_EDGE('',*,*,#13696,.T.);
#18223=ORIENTED_EDGE('',*,*,#13874,.F.);
#18224=ORIENTED_EDGE('',*,*,#13876,.T.);
#18225=ORIENTED_EDGE('',*,*,#13873,.F.);
#18226=ORIENTED_EDGE('',*,*,#13877,.F.);
#18227=ORIENTED_EDGE('',*,*,#13878,.F.);
#18228=ORIENTED_EDGE('',*,*,#13879,.T.);
#18229=ORIENTED_EDGE('',*,*,#13871,.F.);
#18230=ORIENTED_EDGE('',*,*,#13880,.F.);
#18231=ORIENTED_EDGE('',*,*,#13881,.F.);
#18232=ORIENTED_EDGE('',*,*,#13877,.T.);
#18233=ORIENTED_EDGE('',*,*,#13666,.T.);
#18234=ORIENTED_EDGE('',*,*,#13882,.T.);
#18235=ORIENTED_EDGE('',*,*,#13883,.T.);
#18236=ORIENTED_EDGE('',*,*,#13884,.T.);
#18237=ORIENTED_EDGE('',*,*,#13885,.T.);
#18238=ORIENTED_EDGE('',*,*,#13883,.F.);
#18239=ORIENTED_EDGE('',*,*,#13886,.T.);
#18240=ORIENTED_EDGE('',*,*,#13887,.F.);
#18241=ORIENTED_EDGE('',*,*,#13888,.T.);
#18242=ORIENTED_EDGE('',*,*,#13884,.F.);
#18243=ORIENTED_EDGE('',*,*,#13885,.F.);
#18244=ORIENTED_EDGE('',*,*,#13888,.F.);
#18245=ORIENTED_EDGE('',*,*,#13668,.T.);
#18246=ORIENTED_EDGE('',*,*,#13889,.T.);
#18247=ORIENTED_EDGE('',*,*,#13890,.T.);
#18248=ORIENTED_EDGE('',*,*,#13891,.T.);
#18249=ORIENTED_EDGE('',*,*,#13890,.F.);
#18250=ORIENTED_EDGE('',*,*,#13892,.T.);
#18251=ORIENTED_EDGE('',*,*,#13893,.F.);
#18252=ORIENTED_EDGE('',*,*,#13894,.T.);
#18253=ORIENTED_EDGE('',*,*,#13891,.F.);
#18254=ORIENTED_EDGE('',*,*,#13894,.F.);
#18255=ORIENTED_EDGE('',*,*,#13895,.T.);
#18256=ORIENTED_EDGE('',*,*,#13896,.T.);
#18257=ORIENTED_EDGE('',*,*,#13897,.T.);
#18258=ORIENTED_EDGE('',*,*,#13881,.T.);
#18259=ORIENTED_EDGE('',*,*,#13898,.T.);
#18260=ORIENTED_EDGE('',*,*,#13899,.T.);
#18261=ORIENTED_EDGE('',*,*,#13895,.F.);
#18262=ORIENTED_EDGE('',*,*,#13900,.T.);
#18263=ORIENTED_EDGE('',*,*,#13901,.T.);
#18264=ORIENTED_EDGE('',*,*,#13902,.T.);
#18265=ORIENTED_EDGE('',*,*,#13898,.F.);
#18266=ORIENTED_EDGE('',*,*,#13903,.T.);
#18267=ORIENTED_EDGE('',*,*,#13897,.F.);
#18268=ORIENTED_EDGE('',*,*,#13904,.T.);
#18269=ORIENTED_EDGE('',*,*,#13901,.F.);
#18270=ORIENTED_EDGE('',*,*,#13878,.T.);
#18271=ORIENTED_EDGE('',*,*,#13876,.F.);
#18272=ORIENTED_EDGE('',*,*,#13905,.F.);
#18273=ORIENTED_EDGE('',*,*,#13900,.F.);
#18274=ORIENTED_EDGE('',*,*,#13880,.T.);
#18275=ORIENTED_EDGE('',*,*,#13906,.F.);
#18276=ORIENTED_EDGE('',*,*,#13907,.F.);
#18277=ORIENTED_EDGE('',*,*,#13908,.F.);
#18278=ORIENTED_EDGE('',*,*,#13909,.F.);
#18279=ORIENTED_EDGE('',*,*,#13910,.F.);
#18280=ORIENTED_EDGE('',*,*,#13911,.F.);
#18281=ORIENTED_EDGE('',*,*,#13912,.T.);
#18282=ORIENTED_EDGE('',*,*,#13913,.F.);
#18283=ORIENTED_EDGE('',*,*,#13914,.F.);
#18284=ORIENTED_EDGE('',*,*,#13733,.F.);
#18285=ORIENTED_EDGE('',*,*,#13737,.F.);
#18286=ORIENTED_EDGE('',*,*,#13915,.F.);
#18287=ORIENTED_EDGE('',*,*,#13916,.T.);
#18288=ORIENTED_EDGE('',*,*,#13917,.F.);
#18289=ORIENTED_EDGE('',*,*,#13918,.F.);
#18290=ORIENTED_EDGE('',*,*,#13919,.F.);
#18291=ORIENTED_EDGE('',*,*,#13920,.F.);
#18292=ORIENTED_EDGE('',*,*,#13921,.F.);
#18293=ORIENTED_EDGE('',*,*,#13922,.F.);
#18294=ORIENTED_EDGE('',*,*,#13923,.F.);
#18295=ORIENTED_EDGE('',*,*,#13924,.F.);
#18296=ORIENTED_EDGE('',*,*,#13925,.F.);
#18297=ORIENTED_EDGE('',*,*,#13926,.F.);
#18298=ORIENTED_EDGE('',*,*,#13927,.F.);
#18299=ORIENTED_EDGE('',*,*,#13928,.F.);
#18300=ORIENTED_EDGE('',*,*,#13929,.F.);
#18301=ORIENTED_EDGE('',*,*,#13930,.F.);
#18302=ORIENTED_EDGE('',*,*,#13931,.F.);
#18303=ORIENTED_EDGE('',*,*,#13932,.F.);
#18304=ORIENTED_EDGE('',*,*,#13933,.F.);
#18305=ORIENTED_EDGE('',*,*,#13934,.F.);
#18306=ORIENTED_EDGE('',*,*,#13935,.F.);
#18307=ORIENTED_EDGE('',*,*,#13936,.F.);
#18308=ORIENTED_EDGE('',*,*,#13937,.F.);
#18309=ORIENTED_EDGE('',*,*,#13896,.F.);
#18310=ORIENTED_EDGE('',*,*,#13899,.F.);
#18311=ORIENTED_EDGE('',*,*,#13902,.F.);
#18312=ORIENTED_EDGE('',*,*,#13904,.F.);
#18313=ORIENTED_EDGE('',*,*,#13938,.T.);
#18314=ORIENTED_EDGE('',*,*,#13926,.T.);
#18315=ORIENTED_EDGE('',*,*,#13939,.T.);
#18316=ORIENTED_EDGE('',*,*,#13868,.T.);
#18317=ORIENTED_EDGE('',*,*,#13940,.T.);
#18318=ORIENTED_EDGE('',*,*,#13927,.T.);
#18319=ORIENTED_EDGE('',*,*,#13938,.F.);
#18320=ORIENTED_EDGE('',*,*,#13941,.T.);
#18321=ORIENTED_EDGE('',*,*,#13942,.T.);
#18322=ORIENTED_EDGE('',*,*,#13928,.T.);
#18323=ORIENTED_EDGE('',*,*,#13940,.F.);
#18324=ORIENTED_EDGE('',*,*,#13943,.T.);
#18325=ORIENTED_EDGE('',*,*,#13939,.F.);
#18326=ORIENTED_EDGE('',*,*,#13929,.T.);
#18327=ORIENTED_EDGE('',*,*,#13942,.F.);
#18328=ORIENTED_EDGE('',*,*,#13865,.T.);
#18329=ORIENTED_EDGE('',*,*,#13863,.F.);
#18330=ORIENTED_EDGE('',*,*,#13944,.F.);
#18331=ORIENTED_EDGE('',*,*,#13941,.F.);
#18332=ORIENTED_EDGE('',*,*,#13867,.T.);
#18333=ORIENTED_EDGE('',*,*,#13945,.T.);
#18334=ORIENTED_EDGE('',*,*,#13934,.T.);
#18335=ORIENTED_EDGE('',*,*,#13946,.T.);
#18336=ORIENTED_EDGE('',*,*,#13855,.T.);
#18337=ORIENTED_EDGE('',*,*,#13947,.T.);
#18338=ORIENTED_EDGE('',*,*,#13935,.T.);
#18339=ORIENTED_EDGE('',*,*,#13945,.F.);
#18340=ORIENTED_EDGE('',*,*,#13948,.T.);
#18341=ORIENTED_EDGE('',*,*,#13949,.T.);
#18342=ORIENTED_EDGE('',*,*,#13936,.T.);
#18343=ORIENTED_EDGE('',*,*,#13947,.F.);
#18344=ORIENTED_EDGE('',*,*,#13950,.T.);
#18345=ORIENTED_EDGE('',*,*,#13946,.F.);
#18346=ORIENTED_EDGE('',*,*,#13937,.T.);
#18347=ORIENTED_EDGE('',*,*,#13949,.F.);
#18348=ORIENTED_EDGE('',*,*,#13852,.T.);
#18349=ORIENTED_EDGE('',*,*,#13850,.F.);
#18350=ORIENTED_EDGE('',*,*,#13951,.F.);
#18351=ORIENTED_EDGE('',*,*,#13948,.F.);
#18352=ORIENTED_EDGE('',*,*,#13854,.T.);
#18353=ORIENTED_EDGE('',*,*,#13952,.T.);
#18354=ORIENTED_EDGE('',*,*,#13930,.T.);
#18355=ORIENTED_EDGE('',*,*,#13953,.T.);
#18356=ORIENTED_EDGE('',*,*,#13842,.T.);
#18357=ORIENTED_EDGE('',*,*,#13954,.T.);
#18358=ORIENTED_EDGE('',*,*,#13931,.T.);
#18359=ORIENTED_EDGE('',*,*,#13952,.F.);
#18360=ORIENTED_EDGE('',*,*,#13955,.T.);
#18361=ORIENTED_EDGE('',*,*,#13956,.T.);
#18362=ORIENTED_EDGE('',*,*,#13932,.T.);
#18363=ORIENTED_EDGE('',*,*,#13954,.F.);
#18364=ORIENTED_EDGE('',*,*,#13957,.T.);
#18365=ORIENTED_EDGE('',*,*,#13953,.F.);
#18366=ORIENTED_EDGE('',*,*,#13933,.T.);
#18367=ORIENTED_EDGE('',*,*,#13956,.F.);
#18368=ORIENTED_EDGE('',*,*,#13839,.T.);
#18369=ORIENTED_EDGE('',*,*,#13837,.F.);
#18370=ORIENTED_EDGE('',*,*,#13958,.F.);
#18371=ORIENTED_EDGE('',*,*,#13955,.F.);
#18372=ORIENTED_EDGE('',*,*,#13841,.T.);
#18373=ORIENTED_EDGE('',*,*,#13959,.T.);
#18374=ORIENTED_EDGE('',*,*,#13960,.F.);
#18375=ORIENTED_EDGE('',*,*,#13803,.T.);
#18376=ORIENTED_EDGE('',*,*,#13815,.T.);
#18377=ORIENTED_EDGE('',*,*,#13961,.T.);
#18378=ORIENTED_EDGE('',*,*,#13962,.F.);
#18379=ORIENTED_EDGE('',*,*,#13963,.T.);
#18380=ORIENTED_EDGE('',*,*,#13809,.T.);
#18381=ORIENTED_EDGE('',*,*,#13962,.T.);
#18382=ORIENTED_EDGE('',*,*,#13964,.T.);
#18383=ORIENTED_EDGE('',*,*,#13965,.T.);
#18384=ORIENTED_EDGE('',*,*,#13966,.T.);
#18385=ORIENTED_EDGE('',*,*,#13967,.T.);
#18386=ORIENTED_EDGE('',*,*,#13919,.T.);
#18387=ORIENTED_EDGE('',*,*,#13968,.T.);
#18388=ORIENTED_EDGE('',*,*,#13969,.T.);
#18389=ORIENTED_EDGE('',*,*,#13970,.T.);
#18390=ORIENTED_EDGE('',*,*,#13920,.T.);
#18391=ORIENTED_EDGE('',*,*,#13967,.F.);
#18392=ORIENTED_EDGE('',*,*,#13971,.T.);
#18393=ORIENTED_EDGE('',*,*,#13972,.T.);
#18394=ORIENTED_EDGE('',*,*,#13921,.T.);
#18395=ORIENTED_EDGE('',*,*,#13970,.F.);
#18396=ORIENTED_EDGE('',*,*,#13973,.T.);
#18397=ORIENTED_EDGE('',*,*,#13974,.T.);
#18398=ORIENTED_EDGE('',*,*,#13922,.T.);
#18399=ORIENTED_EDGE('',*,*,#13972,.F.);
#18400=ORIENTED_EDGE('',*,*,#13975,.T.);
#18401=ORIENTED_EDGE('',*,*,#13976,.T.);
#18402=ORIENTED_EDGE('',*,*,#13923,.T.);
#18403=ORIENTED_EDGE('',*,*,#13974,.F.);
#18404=ORIENTED_EDGE('',*,*,#13977,.T.);
#18405=ORIENTED_EDGE('',*,*,#13978,.T.);
#18406=ORIENTED_EDGE('',*,*,#13924,.T.);
#18407=ORIENTED_EDGE('',*,*,#13976,.F.);
#18408=ORIENTED_EDGE('',*,*,#13800,.T.);
#18409=ORIENTED_EDGE('',*,*,#13979,.T.);
#18410=ORIENTED_EDGE('',*,*,#13925,.T.);
#18411=ORIENTED_EDGE('',*,*,#13978,.F.);
#18412=ORIENTED_EDGE('',*,*,#13806,.T.);
#18413=ORIENTED_EDGE('',*,*,#13968,.F.);
#18414=ORIENTED_EDGE('',*,*,#13918,.T.);
#18415=ORIENTED_EDGE('',*,*,#13965,.F.);
#18416=ORIENTED_EDGE('',*,*,#13980,.T.);
#18417=ORIENTED_EDGE('',*,*,#13960,.T.);
#18418=ORIENTED_EDGE('',*,*,#13981,.T.);
#18419=ORIENTED_EDGE('',*,*,#13982,.T.);
#18420=ORIENTED_EDGE('',*,*,#13804,.T.);
#18421=ORIENTED_EDGE('',*,*,#13982,.F.);
#18422=ORIENTED_EDGE('',*,*,#13906,.T.);
#18423=ORIENTED_EDGE('',*,*,#13979,.F.);
#18424=ORIENTED_EDGE('',*,*,#13805,.T.);
#18425=ORIENTED_EDGE('',*,*,#13981,.F.);
#18426=ORIENTED_EDGE('',*,*,#13959,.F.);
#18427=ORIENTED_EDGE('',*,*,#13814,.T.);
#18428=ORIENTED_EDGE('',*,*,#13983,.F.);
#18429=ORIENTED_EDGE('',*,*,#13907,.T.);
#18430=ORIENTED_EDGE('',*,*,#13777,.F.);
#18431=ORIENTED_EDGE('',*,*,#13801,.T.);
#18432=ORIENTED_EDGE('',*,*,#13977,.F.);
#18433=ORIENTED_EDGE('',*,*,#13984,.F.);
#18434=ORIENTED_EDGE('',*,*,#13774,.F.);
#18435=ORIENTED_EDGE('',*,*,#13984,.T.);
#18436=ORIENTED_EDGE('',*,*,#13975,.F.);
#18437=ORIENTED_EDGE('',*,*,#13985,.F.);
#18438=ORIENTED_EDGE('',*,*,#13771,.F.);
#18439=ORIENTED_EDGE('',*,*,#13985,.T.);
#18440=ORIENTED_EDGE('',*,*,#13973,.F.);
#18441=ORIENTED_EDGE('',*,*,#13986,.F.);
#18442=ORIENTED_EDGE('',*,*,#13768,.F.);
#18443=ORIENTED_EDGE('',*,*,#13986,.T.);
#18444=ORIENTED_EDGE('',*,*,#13971,.F.);
#18445=ORIENTED_EDGE('',*,*,#13987,.F.);
#18446=ORIENTED_EDGE('',*,*,#13702,.F.);
#18447=ORIENTED_EDGE('',*,*,#13706,.F.);
#18448=ORIENTED_EDGE('',*,*,#13787,.F.);
#18449=ORIENTED_EDGE('',*,*,#13782,.F.);
#18450=ORIENTED_EDGE('',*,*,#13988,.T.);
#18451=ORIENTED_EDGE('',*,*,#13911,.T.);
#18452=ORIENTED_EDGE('',*,*,#13989,.T.);
#18453=ORIENTED_EDGE('',*,*,#13990,.T.);
#18454=ORIENTED_EDGE('',*,*,#13991,.T.);
#18455=ORIENTED_EDGE('',*,*,#13992,.T.);
#18456=ORIENTED_EDGE('',*,*,#13993,.T.);
#18457=ORIENTED_EDGE('',*,*,#13990,.F.);
#18458=ORIENTED_EDGE('',*,*,#13994,.T.);
#18459=ORIENTED_EDGE('',*,*,#13995,.T.);
#18460=ORIENTED_EDGE('',*,*,#13996,.T.);
#18461=ORIENTED_EDGE('',*,*,#13997,.T.);
#18462=ORIENTED_EDGE('',*,*,#13994,.F.);
#18463=ORIENTED_EDGE('',*,*,#13998,.T.);
#18464=ORIENTED_EDGE('',*,*,#13992,.F.);
#18465=ORIENTED_EDGE('',*,*,#13999,.T.);
#18466=ORIENTED_EDGE('',*,*,#13739,.F.);
#18467=ORIENTED_EDGE('',*,*,#14000,.T.);
#18468=ORIENTED_EDGE('',*,*,#13996,.F.);
#18469=ORIENTED_EDGE('',*,*,#14001,.T.);
#18470=ORIENTED_EDGE('',*,*,#13988,.F.);
#18471=ORIENTED_EDGE('',*,*,#13993,.F.);
#18472=ORIENTED_EDGE('',*,*,#13998,.F.);
#18473=ORIENTED_EDGE('',*,*,#14002,.T.);
#18474=ORIENTED_EDGE('',*,*,#14003,.F.);
#18475=ORIENTED_EDGE('',*,*,#13912,.F.);
#18476=ORIENTED_EDGE('',*,*,#13997,.F.);
#18477=ORIENTED_EDGE('',*,*,#14004,.T.);
#18478=ORIENTED_EDGE('',*,*,#14005,.F.);
#18479=ORIENTED_EDGE('',*,*,#14002,.F.);
#18480=ORIENTED_EDGE('',*,*,#13734,.F.);
#18481=ORIENTED_EDGE('',*,*,#13914,.T.);
#18482=ORIENTED_EDGE('',*,*,#14006,.F.);
#18483=ORIENTED_EDGE('',*,*,#14004,.F.);
#18484=ORIENTED_EDGE('',*,*,#14000,.F.);
#18485=ORIENTED_EDGE('',*,*,#13738,.F.);
#18486=ORIENTED_EDGE('',*,*,#14007,.T.);
#18487=ORIENTED_EDGE('',*,*,#13909,.T.);
#18488=ORIENTED_EDGE('',*,*,#14008,.T.);
#18489=ORIENTED_EDGE('',*,*,#14009,.T.);
#18490=ORIENTED_EDGE('',*,*,#14010,.T.);
#18491=ORIENTED_EDGE('',*,*,#14011,.T.);
#18492=ORIENTED_EDGE('',*,*,#13723,.T.);
#18493=ORIENTED_EDGE('',*,*,#14012,.T.);
#18494=ORIENTED_EDGE('',*,*,#14009,.F.);
#18495=ORIENTED_EDGE('',*,*,#13989,.F.);
#18496=ORIENTED_EDGE('',*,*,#13910,.T.);
#18497=ORIENTED_EDGE('',*,*,#14007,.F.);
#18498=ORIENTED_EDGE('',*,*,#14013,.T.);
#18499=ORIENTED_EDGE('',*,*,#13991,.F.);
#18500=ORIENTED_EDGE('',*,*,#14013,.F.);
#18501=ORIENTED_EDGE('',*,*,#14010,.F.);
#18502=ORIENTED_EDGE('',*,*,#14012,.F.);
#18503=ORIENTED_EDGE('',*,*,#13722,.F.);
#18504=ORIENTED_EDGE('',*,*,#14014,.F.);
#18505=ORIENTED_EDGE('',*,*,#14015,.F.);
#18506=ORIENTED_EDGE('',*,*,#13735,.F.);
#18507=ORIENTED_EDGE('',*,*,#13740,.F.);
#18508=ORIENTED_EDGE('',*,*,#14001,.F.);
#18509=ORIENTED_EDGE('',*,*,#13995,.F.);
#18510=ORIENTED_EDGE('',*,*,#13999,.F.);
#18511=ORIENTED_EDGE('',*,*,#14016,.T.);
#18512=ORIENTED_EDGE('',*,*,#13915,.T.);
#18513=ORIENTED_EDGE('',*,*,#13736,.T.);
#18514=ORIENTED_EDGE('',*,*,#14015,.T.);
#18515=ORIENTED_EDGE('',*,*,#14017,.T.);
#18516=ORIENTED_EDGE('',*,*,#14014,.T.);
#18517=ORIENTED_EDGE('',*,*,#13721,.T.);
#18518=ORIENTED_EDGE('',*,*,#14018,.T.);
#18519=ORIENTED_EDGE('',*,*,#14017,.F.);
#18520=ORIENTED_EDGE('',*,*,#14016,.F.);
#18521=ORIENTED_EDGE('',*,*,#14018,.F.);
#18522=ORIENTED_EDGE('',*,*,#13720,.F.);
#18523=ORIENTED_EDGE('',*,*,#14019,.F.);
#18524=ORIENTED_EDGE('',*,*,#14020,.F.);
#18525=ORIENTED_EDGE('',*,*,#13916,.F.);
#18526=ORIENTED_EDGE('',*,*,#14021,.T.);
#18527=ORIENTED_EDGE('',*,*,#13811,.T.);
#18528=ORIENTED_EDGE('',*,*,#14022,.T.);
#18529=ORIENTED_EDGE('',*,*,#14020,.T.);
#18530=ORIENTED_EDGE('',*,*,#13727,.T.);
#18531=ORIENTED_EDGE('',*,*,#14023,.T.);
#18532=ORIENTED_EDGE('',*,*,#14021,.F.);
#18533=ORIENTED_EDGE('',*,*,#14019,.T.);
#18534=ORIENTED_EDGE('',*,*,#14024,.T.);
#18535=ORIENTED_EDGE('',*,*,#14025,.T.);
#18536=ORIENTED_EDGE('',*,*,#13725,.T.);
#18537=ORIENTED_EDGE('',*,*,#14026,.T.);
#18538=ORIENTED_EDGE('',*,*,#13983,.T.);
#18539=ORIENTED_EDGE('',*,*,#13813,.T.);
#18540=ORIENTED_EDGE('',*,*,#14024,.F.);
#18541=ORIENTED_EDGE('',*,*,#14027,.T.);
#18542=ORIENTED_EDGE('',*,*,#14008,.F.);
#18543=ORIENTED_EDGE('',*,*,#13908,.T.);
#18544=ORIENTED_EDGE('',*,*,#14027,.F.);
#18545=ORIENTED_EDGE('',*,*,#14026,.F.);
#18546=ORIENTED_EDGE('',*,*,#13724,.F.);
#18547=ORIENTED_EDGE('',*,*,#14011,.F.);
#18548=ORIENTED_EDGE('',*,*,#14003,.T.);
#18549=ORIENTED_EDGE('',*,*,#14028,.T.);
#18550=ORIENTED_EDGE('',*,*,#13816,.T.);
#18551=ORIENTED_EDGE('',*,*,#14029,.T.);
#18552=ORIENTED_EDGE('',*,*,#13913,.T.);
#18553=ORIENTED_EDGE('',*,*,#14029,.F.);
#18554=ORIENTED_EDGE('',*,*,#13819,.T.);
#18555=ORIENTED_EDGE('',*,*,#14030,.T.);
#18556=ORIENTED_EDGE('',*,*,#14031,.T.);
#18557=ORIENTED_EDGE('',*,*,#13817,.T.);
#18558=ORIENTED_EDGE('',*,*,#14028,.F.);
#18559=ORIENTED_EDGE('',*,*,#14005,.T.);
#18560=ORIENTED_EDGE('',*,*,#13818,.T.);
#18561=ORIENTED_EDGE('',*,*,#14031,.F.);
#18562=ORIENTED_EDGE('',*,*,#14006,.T.);
#18563=ORIENTED_EDGE('',*,*,#14030,.F.);
#18564=ORIENTED_EDGE('',*,*,#13966,.F.);
#18565=ORIENTED_EDGE('',*,*,#13917,.T.);
#18566=ORIENTED_EDGE('',*,*,#14022,.F.);
#18567=ORIENTED_EDGE('',*,*,#13810,.T.);
#18568=ORIENTED_EDGE('',*,*,#13963,.F.);
#18569=ORIENTED_EDGE('',*,*,#13790,.F.);
#18570=ORIENTED_EDGE('',*,*,#13987,.T.);
#18571=ORIENTED_EDGE('',*,*,#13969,.F.);
#18572=ORIENTED_EDGE('',*,*,#13980,.F.);
#18573=ORIENTED_EDGE('',*,*,#13964,.F.);
#18574=ORIENTED_EDGE('',*,*,#13961,.F.);
#18575=ORIENTED_EDGE('',*,*,#13808,.F.);
#18576=ORIENTED_EDGE('',*,*,#13747,.F.);
#18577=ORIENTED_EDGE('',*,*,#13751,.F.);
#18578=ORIENTED_EDGE('',*,*,#13794,.F.);
#18579=ORIENTED_EDGE('',*,*,#14023,.F.);
#18580=ORIENTED_EDGE('',*,*,#13726,.T.);
#18581=ORIENTED_EDGE('',*,*,#14025,.F.);
#18582=ORIENTED_EDGE('',*,*,#13812,.T.);
#18583=ORIENTED_EDGE('',*,*,#13875,.F.);
#18584=ORIENTED_EDGE('',*,*,#13879,.F.);
#18585=ORIENTED_EDGE('',*,*,#13903,.F.);
#18586=ORIENTED_EDGE('',*,*,#13905,.T.);
#18587=ORIENTED_EDGE('',*,*,#13862,.F.);
#18588=ORIENTED_EDGE('',*,*,#13866,.F.);
#18589=ORIENTED_EDGE('',*,*,#13943,.F.);
#18590=ORIENTED_EDGE('',*,*,#13944,.T.);
#18591=ORIENTED_EDGE('',*,*,#13849,.F.);
#18592=ORIENTED_EDGE('',*,*,#13853,.F.);
#18593=ORIENTED_EDGE('',*,*,#13950,.F.);
#18594=ORIENTED_EDGE('',*,*,#13951,.T.);
#18595=ORIENTED_EDGE('',*,*,#13836,.F.);
#18596=ORIENTED_EDGE('',*,*,#13840,.F.);
#18597=ORIENTED_EDGE('',*,*,#13957,.F.);
#18598=ORIENTED_EDGE('',*,*,#13958,.T.);
#18599=ORIENTED_EDGE('',*,*,#14032,.T.);
#18600=ORIENTED_EDGE('',*,*,#13678,.T.);
#18601=ORIENTED_EDGE('',*,*,#14032,.F.);
#18602=ORIENTED_EDGE('',*,*,#14033,.T.);
#18603=ORIENTED_EDGE('',*,*,#13893,.T.);
#18604=ORIENTED_EDGE('',*,*,#14033,.F.);
#18605=ORIENTED_EDGE('',*,*,#14034,.T.);
#18606=ORIENTED_EDGE('',*,*,#13887,.T.);
#18607=ORIENTED_EDGE('',*,*,#14034,.F.);
#18608=ORIENTED_EDGE('',*,*,#14035,.T.);
#18609=ORIENTED_EDGE('',*,*,#13672,.T.);
#18610=ORIENTED_EDGE('',*,*,#14035,.F.);
#18611=ORIENTED_EDGE('',*,*,#13729,.F.);
#18612=ORIENTED_EDGE('',*,*,#14036,.T.);
#18613=ORIENTED_EDGE('',*,*,#14036,.F.);
#18614=ORIENTED_EDGE('',*,*,#14037,.T.);
#18615=ORIENTED_EDGE('',*,*,#14038,.F.);
#18616=ORIENTED_EDGE('',*,*,#14039,.F.);
#18617=ORIENTED_EDGE('',*,*,#14037,.F.);
#18618=ORIENTED_EDGE('',*,*,#14040,.F.);
#18619=ORIENTED_EDGE('',*,*,#14041,.F.);
#18620=ORIENTED_EDGE('',*,*,#14042,.T.);
#18621=ORIENTED_EDGE('',*,*,#14043,.T.);
#18622=ORIENTED_EDGE('',*,*,#14042,.F.);
#18623=ORIENTED_EDGE('',*,*,#14043,.F.);
#18624=ORIENTED_EDGE('',*,*,#14044,.T.);
#18625=ORIENTED_EDGE('',*,*,#14044,.F.);
#18626=ORIENTED_EDGE('',*,*,#14045,.T.);
#18627=ORIENTED_EDGE('',*,*,#13648,.F.);
#18628=ORIENTED_EDGE('',*,*,#14045,.F.);
#18629=ORIENTED_EDGE('',*,*,#14046,.F.);
#18630=ORIENTED_EDGE('',*,*,#14047,.T.);
#18631=ORIENTED_EDGE('',*,*,#13712,.F.);
#18632=ORIENTED_EDGE('',*,*,#14047,.F.);
#18633=ORIENTED_EDGE('',*,*,#14038,.T.);
#18634=ORIENTED_EDGE('',*,*,#14039,.T.);
#18635=ORIENTED_EDGE('',*,*,#14040,.T.);
#18636=ORIENTED_EDGE('',*,*,#14041,.T.);
#18637=ORIENTED_EDGE('',*,*,#13656,.F.);
#18638=ORIENTED_EDGE('',*,*,#13664,.F.);
#18639=ORIENTED_EDGE('',*,*,#13671,.F.);
#18640=ORIENTED_EDGE('',*,*,#13677,.F.);
#18641=ORIENTED_EDGE('',*,*,#13674,.F.);
#18642=ORIENTED_EDGE('',*,*,#13669,.F.);
#18643=ORIENTED_EDGE('',*,*,#13892,.F.);
#18644=ORIENTED_EDGE('',*,*,#13889,.F.);
#18645=ORIENTED_EDGE('',*,*,#13667,.F.);
#18646=ORIENTED_EDGE('',*,*,#13886,.F.);
#18647=ORIENTED_EDGE('',*,*,#13882,.F.);
#18648=ORIENTED_EDGE('',*,*,#13665,.F.);
#18649=ORIENTED_EDGE('',*,*,#13660,.F.);
#18650=ORIENTED_EDGE('',*,*,#14046,.T.);
#24967=CONICAL_SURFACE('',#27142,1.69267766952967,1.17809724509617);
#24968=CONICAL_SURFACE('',#27146,1.75,0.785398163397413);
#24969=CONICAL_SURFACE('',#27151,1.78232233047033,0.39269908169871);
#24970=CONICAL_SURFACE('',#27155,0.330000000000001,0.785398163397462);
#24971=CONICAL_SURFACE('',#27160,5.4,0.785398163397451);
#24972=CONICAL_SURFACE('',#27170,0.329999999999999,0.785398163397428);
#24973=CONICAL_SURFACE('',#27186,5.29267766952966,1.17809724509617);
#24974=CONICAL_SURFACE('',#27189,5.4,0.785398163397442);
#24975=CONICAL_SURFACE('',#27199,5.48232233047034,0.392699081698728);
#24976=CONICAL_SURFACE('',#27202,19.3603883884215,0.785398163397445);
#24977=CONICAL_SURFACE('',#27211,0.975,0.785398163397449);
#24978=CONICAL_SURFACE('',#27215,0.975,0.785398163397449);
#24979=CONICAL_SURFACE('',#27223,0.975,0.785398163397454);
#24980=CONICAL_SURFACE('',#27225,0.975000000000002,0.785398163397454);
#24981=CONICAL_SURFACE('',#27243,0.575000000000001,0.785398163397457);
#24982=CONICAL_SURFACE('',#27246,0.575000000000001,0.785398163397457);
#24983=CONICAL_SURFACE('',#27252,0.575000000000001,0.785398163397457);
#24984=CONICAL_SURFACE('',#27255,0.575000000000001,0.785398163397457);
#24985=CONICAL_SURFACE('',#27261,0.575000000000001,0.785398163397457);
#24986=CONICAL_SURFACE('',#27264,0.575000000000001,0.785398163397457);
#24987=CONICAL_SURFACE('',#27270,0.575000000000001,0.785398163397457);
#24988=CONICAL_SURFACE('',#27273,0.575000000000001,0.785398163397457);
#24989=CONICAL_SURFACE('',#27278,0.330000000000001,0.785398163397462);
#24990=CONICAL_SURFACE('',#27285,0.33,0.785398163397456);
#24991=CONICAL_SURFACE('',#27292,0.575000000000001,0.785398163397457);
#24992=CONICAL_SURFACE('',#27296,0.575000000000001,0.785398163397457);
#24993=CONICAL_SURFACE('',#27311,0.575000000000001,0.785398163397457);
#24994=CONICAL_SURFACE('',#27314,0.575000000000001,0.785398163397457);
#24995=CONICAL_SURFACE('',#27317,0.575000000000001,0.785398163397457);
#24996=CONICAL_SURFACE('',#27320,0.575000000000001,0.785398163397457);
#24997=CONICAL_SURFACE('',#27323,0.575000000000001,0.785398163397457);
#24998=CONICAL_SURFACE('',#27326,0.575000000000001,0.785398163397457);
#24999=CONICAL_SURFACE('',#27328,0.975,0.785398163397454);
#25000=CONICAL_SURFACE('',#27331,0.975,0.785398163397449);
#25001=CONICAL_SURFACE('',#27334,0.975,0.785398163397449);
#25002=CONICAL_SURFACE('',#27337,0.975000000000002,0.785398163397454);
#25003=CONICAL_SURFACE('',#27345,19.3603883884215,0.785398163397445);
#25004=CONICAL_SURFACE('',#27380,0.1525,1.02974425867665);
#25005=CONICAL_SURFACE('',#27381,0.1525,1.02974425867665);
#25006=CONICAL_SURFACE('',#27382,0.1525,1.02974425867665);
#25007=CONICAL_SURFACE('',#27383,0.1525,1.02974425867665);
#25258=ADVANCED_FACE('',(#2670),#24967,.T.);
#25259=ADVANCED_FACE('',(#2671),#24968,.T.);
#25260=ADVANCED_FACE('',(#2672,#1561),#1737,.T.);
#25261=ADVANCED_FACE('',(#2673),#24969,.T.);
#25262=ADVANCED_FACE('',(#2674),#1122,.T.);
#25263=ADVANCED_FACE('',(#2675),#24970,.F.);
#25264=ADVANCED_FACE('',(#2676),#24971,.T.);
#25265=ADVANCED_FACE('',(#2677),#1123,.F.);
#25266=ADVANCED_FACE('',(#2678),#24972,.F.);
#25267=ADVANCED_FACE('',(#2679),#1124,.F.);
#25268=ADVANCED_FACE('',(#2680),#1738,.T.);
#25269=ADVANCED_FACE('',(#2681,#1562,#1563),#1739,.F.);
#25270=ADVANCED_FACE('',(#2682),#1740,.T.);
#25271=ADVANCED_FACE('',(#2683),#1741,.T.);
#25272=ADVANCED_FACE('',(#2684),#24973,.T.);
#25273=ADVANCED_FACE('',(#2685),#24974,.T.);
#25274=ADVANCED_FACE('',(#2686,#1564),#1742,.T.);
#25275=ADVANCED_FACE('',(#2687),#138,.T.);
#25276=ADVANCED_FACE('',(#2688,#1565,#1566,#1567),#1125,.T.);
#25277=ADVANCED_FACE('',(#2689),#1126,.F.);
#25278=ADVANCED_FACE('',(#2690),#24975,.T.);
#25279=ADVANCED_FACE('',(#2691),#1743,.T.);
#25280=ADVANCED_FACE('',(#2692),#1744,.F.);
#25281=ADVANCED_FACE('',(#2693),#24976,.T.);
#25282=ADVANCED_FACE('',(#2694),#139,.T.);
#25283=ADVANCED_FACE('',(#2695),#140,.T.);
#25284=ADVANCED_FACE('',(#2696),#141,.T.);
#25285=ADVANCED_FACE('',(#2697),#1745,.T.);
#25286=ADVANCED_FACE('',(#2698),#1746,.T.);
#25287=ADVANCED_FACE('',(#2699),#1747,.T.);
#25288=ADVANCED_FACE('',(#2700),#1748,.T.);
#25289=ADVANCED_FACE('',(#2701),#1749,.T.);
#25290=ADVANCED_FACE('',(#2702),#1750,.T.);
#25291=ADVANCED_FACE('',(#2703),#24977,.T.);
#25292=ADVANCED_FACE('',(#2704),#1751,.T.);
#25293=ADVANCED_FACE('',(#2705),#24978,.T.);
#25294=ADVANCED_FACE('',(#2706),#1752,.T.);
#25295=ADVANCED_FACE('',(#2707),#1753,.T.);
#25296=ADVANCED_FACE('',(#2708),#1754,.T.);
#25297=ADVANCED_FACE('',(#2709),#1755,.T.);
#25298=ADVANCED_FACE('',(#2710),#1756,.T.);
#25299=ADVANCED_FACE('',(#2711),#24979,.T.);
#25300=ADVANCED_FACE('',(#2712),#24980,.T.);
#25301=ADVANCED_FACE('',(#2713),#142,.T.);
#25302=ADVANCED_FACE('',(#2714),#143,.T.);
#25303=ADVANCED_FACE('',(#2715),#144,.T.);
#25304=ADVANCED_FACE('',(#2716),#1757,.T.);
#25305=ADVANCED_FACE('',(#2717),#1127,.T.);
#25306=ADVANCED_FACE('',(#2718,#1568),#1758,.T.);
#25307=ADVANCED_FACE('',(#2719),#1128,.T.);
#25308=ADVANCED_FACE('',(#2720),#1759,.F.);
#25309=ADVANCED_FACE('',(#2721),#1760,.F.);
#25310=ADVANCED_FACE('',(#2722),#1761,.F.);
#25311=ADVANCED_FACE('',(#2723,#1569,#1570),#1762,.F.);
#25312=ADVANCED_FACE('',(#2724),#1763,.T.);
#25313=ADVANCED_FACE('',(#2725),#24981,.F.);
#25314=ADVANCED_FACE('',(#2726),#1764,.T.);
#25315=ADVANCED_FACE('',(#2727),#24982,.F.);
#25316=ADVANCED_FACE('',(#2728),#1129,.F.);
#25317=ADVANCED_FACE('',(#2729),#1765,.F.);
#25318=ADVANCED_FACE('',(#2730),#1766,.T.);
#25319=ADVANCED_FACE('',(#2731),#24983,.F.);
#25320=ADVANCED_FACE('',(#2732),#1767,.T.);
#25321=ADVANCED_FACE('',(#2733),#24984,.F.);
#25322=ADVANCED_FACE('',(#2734),#1130,.F.);
#25323=ADVANCED_FACE('',(#2735),#1768,.F.);
#25324=ADVANCED_FACE('',(#2736),#1769,.T.);
#25325=ADVANCED_FACE('',(#2737),#24985,.F.);
#25326=ADVANCED_FACE('',(#2738),#1770,.T.);
#25327=ADVANCED_FACE('',(#2739),#24986,.F.);
#25328=ADVANCED_FACE('',(#2740),#1131,.F.);
#25329=ADVANCED_FACE('',(#2741),#1771,.F.);
#25330=ADVANCED_FACE('',(#2742),#1772,.T.);
#25331=ADVANCED_FACE('',(#2743),#24987,.F.);
#25332=ADVANCED_FACE('',(#2744),#1773,.T.);
#25333=ADVANCED_FACE('',(#2745),#24988,.F.);
#25334=ADVANCED_FACE('',(#2746),#1132,.F.);
#25335=ADVANCED_FACE('',(#2747),#1774,.F.);
#25336=ADVANCED_FACE('',(#2748),#24989,.F.);
#25337=ADVANCED_FACE('',(#2749),#1133,.F.);
#25338=ADVANCED_FACE('',(#2750),#24990,.F.);
#25339=ADVANCED_FACE('',(#2751),#1134,.F.);
#25340=ADVANCED_FACE('',(#2752),#1775,.T.);
#25341=ADVANCED_FACE('',(#2753),#24991,.F.);
#25342=ADVANCED_FACE('',(#2754),#1776,.T.);
#25343=ADVANCED_FACE('',(#2755),#24992,.F.);
#25344=ADVANCED_FACE('',(#2756),#1135,.F.);
#25345=ADVANCED_FACE('',(#2757,#1571,#1572,#1573,#1574),#1777,.T.);
#25346=ADVANCED_FACE('',(#2758),#1778,.T.);
#25347=ADVANCED_FACE('',(#2759),#24993,.F.);
#25348=ADVANCED_FACE('',(#2760),#1779,.T.);
#25349=ADVANCED_FACE('',(#2761),#24994,.F.);
#25350=ADVANCED_FACE('',(#2762),#1136,.F.);
#25351=ADVANCED_FACE('',(#2763),#1780,.T.);
#25352=ADVANCED_FACE('',(#2764),#24995,.F.);
#25353=ADVANCED_FACE('',(#2765),#1781,.T.);
#25354=ADVANCED_FACE('',(#2766),#24996,.F.);
#25355=ADVANCED_FACE('',(#2767),#1137,.F.);
#25356=ADVANCED_FACE('',(#2768),#1782,.T.);
#25357=ADVANCED_FACE('',(#2769),#24997,.F.);
#25358=ADVANCED_FACE('',(#2770),#1783,.T.);
#25359=ADVANCED_FACE('',(#2771),#24998,.F.);
#25360=ADVANCED_FACE('',(#2772),#1138,.F.);
#25361=ADVANCED_FACE('',(#2773),#145,.T.);
#25362=ADVANCED_FACE('',(#2774),#146,.T.);
#25363=ADVANCED_FACE('',(#2775),#147,.T.);
#25364=ADVANCED_FACE('',(#2776),#24999,.T.);
#25365=ADVANCED_FACE('',(#2777),#1784,.T.);
#25366=ADVANCED_FACE('',(#2778),#25000,.T.);
#25367=ADVANCED_FACE('',(#2779),#1785,.T.);
#25368=ADVANCED_FACE('',(#2780),#25001,.T.);
#25369=ADVANCED_FACE('',(#2781),#1786,.T.);
#25370=ADVANCED_FACE('',(#2782),#25002,.T.);
#25371=ADVANCED_FACE('',(#2783),#148,.T.);
#25372=ADVANCED_FACE('',(#2784),#149,.T.);
#25373=ADVANCED_FACE('',(#2785),#150,.T.);
#25374=ADVANCED_FACE('',(#2786),#1139,.T.);
#25375=ADVANCED_FACE('',(#2787),#1140,.T.);
#25376=ADVANCED_FACE('',(#2788),#1787,.T.);
#25377=ADVANCED_FACE('',(#2789),#1141,.T.);
#25378=ADVANCED_FACE('',(#2790),#1788,.T.);
#25379=ADVANCED_FACE('',(#2791),#1789,.T.);
#25380=ADVANCED_FACE('',(#2792),#25003,.T.);
#25381=ADVANCED_FACE('',(#2793),#151,.T.);
#25382=ADVANCED_FACE('',(#2794),#152,.T.);
#25383=ADVANCED_FACE('',(#2795),#153,.T.);
#25384=ADVANCED_FACE('',(#2796),#1790,.T.);
#25385=ADVANCED_FACE('',(#2797),#1142,.F.);
#25386=ADVANCED_FACE('',(#2798),#1791,.T.);
#25387=ADVANCED_FACE('',(#2799),#1792,.T.);
#25388=ADVANCED_FACE('',(#2800),#154,.T.);
#25389=ADVANCED_FACE('',(#2801),#1793,.F.);
#25390=ADVANCED_FACE('',(#2802),#1143,.T.);
#25391=ADVANCED_FACE('',(#2803),#1794,.T.);
#25392=ADVANCED_FACE('',(#2804),#155,.T.);
#25393=ADVANCED_FACE('',(#2805),#1795,.T.);
#25394=ADVANCED_FACE('',(#2806),#1144,.T.);
#25395=ADVANCED_FACE('',(#2807),#156,.F.);
#25396=ADVANCED_FACE('',(#2808),#157,.F.);
#25397=ADVANCED_FACE('',(#2809),#1145,.T.);
#25398=ADVANCED_FACE('',(#2810),#1796,.T.);
#25399=ADVANCED_FACE('',(#2811),#1146,.T.);
#25400=ADVANCED_FACE('',(#2812),#1147,.T.);
#25401=ADVANCED_FACE('',(#2813),#1083,.T.);
#25402=ADVANCED_FACE('',(#2814),#1148,.T.);
#25403=ADVANCED_FACE('',(#2815),#1149,.T.);
#25404=ADVANCED_FACE('',(#2816),#1150,.T.);
#25405=ADVANCED_FACE('',(#2817),#1084,.F.);
#25406=ADVANCED_FACE('',(#2818),#1797,.F.);
#25407=ADVANCED_FACE('',(#2819),#1798,.F.);
#25408=ADVANCED_FACE('',(#2820),#1799,.F.);
#25409=ADVANCED_FACE('',(#2821),#1800,.F.);
#25410=ADVANCED_FACE('',(#2822),#25004,.F.);
#25411=ADVANCED_FACE('',(#2823),#25005,.F.);
#25412=ADVANCED_FACE('',(#2824),#25006,.F.);
#25413=ADVANCED_FACE('',(#2825),#25007,.F.);
#25414=ADVANCED_FACE('',(#2826,#1575),#1801,.F.);
#25415=ADVANCED_FACE('',(#2827),#1151,.F.);
#25416=ADVANCED_FACE('',(#2828),#1152,.F.);
#25417=ADVANCED_FACE('',(#2829,#1576),#1802,.F.);
#25418=ADVANCED_FACE('',(#2830),#1153,.F.);
#25419=ADVANCED_FACE('',(#2831,#1577,#1578),#1154,.F.);
#25420=ADVANCED_FACE('',(#2832,#1579),#1803,.T.);
#26665=CLOSED_SHELL('',(#25258,#25259,#25260,#25261,#25262,#25263,#25264,
#25265,#25266,#25267,#25268,#25269,#25270,#25271,#25272,#25273,#25274,#25275,
#25276,#25277,#25278,#25279,#25280,#25281,#25282,#25283,#25284,#25285,#25286,
#25287,#25288,#25289,#25290,#25291,#25292,#25293,#25294,#25295,#25296,#25297,
#25298,#25299,#25300,#25301,#25302,#25303,#25304,#25305,#25306,#25307,#25308,
#25309,#25310,#25311,#25312,#25313,#25314,#25315,#25316,#25317,#25318,#25319,
#25320,#25321,#25322,#25323,#25324,#25325,#25326,#25327,#25328,#25329,#25330,
#25331,#25332,#25333,#25334,#25335,#25336,#25337,#25338,#25339,#25340,#25341,
#25342,#25343,#25344,#25345,#25346,#25347,#25348,#25349,#25350,#25351,#25352,
#25353,#25354,#25355,#25356,#25357,#25358,#25359,#25360,#25361,#25362,#25363,
#25364,#25365,#25366,#25367,#25368,#25369,#25370,#25371,#25372,#25373,#25374,
#25375,#25376,#25377,#25378,#25379,#25380,#25381,#25382,#25383,#25384,#25385,
#25386,#25387,#25388,#25389,#25390,#25391,#25392,#25393,#25394,#25395,#25396,
#25397,#25398,#25399,#25400,#25401,#25402,#25403,#25404,#25405,#25406,#25407,
#25408,#25409,#25410,#25411,#25412,#25413,#25414,#25415,#25416,#25417,#25418,
#25419,#25420));
#27141=AXIS2_PLACEMENT_3D('',#37039,#30055,#30056);
#27142=AXIS2_PLACEMENT_3D('',#37040,#30057,#30058);
#27143=AXIS2_PLACEMENT_3D('',#37042,#30059,#30060);
#27144=AXIS2_PLACEMENT_3D('',#37046,#30062,#30063);
#27145=AXIS2_PLACEMENT_3D('',#37047,#30064,#30065);
#27146=AXIS2_PLACEMENT_3D('',#37048,#30066,#30067);
#27147=AXIS2_PLACEMENT_3D('',#37052,#30069,#30070);
#27148=AXIS2_PLACEMENT_3D('',#37053,#30071,#30072);
#27149=AXIS2_PLACEMENT_3D('',#37054,#30073,#30074);
#27150=AXIS2_PLACEMENT_3D('',#37056,#30075,#30076);
#27151=AXIS2_PLACEMENT_3D('',#37057,#30077,#30078);
#27152=AXIS2_PLACEMENT_3D('',#37061,#30080,#30081);
#27153=AXIS2_PLACEMENT_3D('',#37062,#30082,#30083);
#27154=AXIS2_PLACEMENT_3D('',#37063,#30084,#30085);
#27155=AXIS2_PLACEMENT_3D('',#37135,#30087,#30088);
#27156=AXIS2_PLACEMENT_3D('',#37145,#30089,#30090);
#27157=AXIS2_PLACEMENT_3D('',#37149,#30092,#30093);
#27158=AXIS2_PLACEMENT_3D('',#37150,#30094,#30095);
#27159=AXIS2_PLACEMENT_3D('',#37151,#30096,#30097);
#27160=AXIS2_PLACEMENT_3D('',#37152,#30098,#30099);
#27161=AXIS2_PLACEMENT_3D('',#37155,#30100,#30101);
#27162=AXIS2_PLACEMENT_3D('',#37156,#30102,#30103);
#27163=AXIS2_PLACEMENT_3D('',#37159,#30105,#30106);
#27164=AXIS2_PLACEMENT_3D('',#37161,#30107,#30108);
#27165=AXIS2_PLACEMENT_3D('',#37170,#30109,#30110);
#27166=AXIS2_PLACEMENT_3D('',#37179,#30111,#30112);
#27167=AXIS2_PLACEMENT_3D('',#37187,#30113,#30114);
#27168=AXIS2_PLACEMENT_3D('',#37188,#30115,#30116);
#27169=AXIS2_PLACEMENT_3D('',#37190,#30117,#30118);
#27170=AXIS2_PLACEMENT_3D('',#37192,#30120,#30121);
#27171=AXIS2_PLACEMENT_3D('',#37194,#30122,#30123);
#27172=AXIS2_PLACEMENT_3D('',#37197,#30125,#30126);
#27173=AXIS2_PLACEMENT_3D('',#37198,#30127,#30128);
#27174=AXIS2_PLACEMENT_3D('',#37199,#30129,#30130);
#27175=AXIS2_PLACEMENT_3D('',#37201,#30131,#30132);
#27176=AXIS2_PLACEMENT_3D('',#37203,#30134,#30135);
#27177=AXIS2_PLACEMENT_3D('',#37216,#30142,#30143);
#27178=AXIS2_PLACEMENT_3D('',#37220,#30145,#30146);
#27179=AXIS2_PLACEMENT_3D('',#37234,#30148,#30149);
#27180=AXIS2_PLACEMENT_3D('',#37240,#30152,#30153);
#27181=AXIS2_PLACEMENT_3D('',#37243,#30155,#30156);
#27182=AXIS2_PLACEMENT_3D('',#37248,#30158,#30159);
#27183=AXIS2_PLACEMENT_3D('',#37251,#30161,#30162);
#27184=AXIS2_PLACEMENT_3D('',#37252,#30163,#30164);
#27185=AXIS2_PLACEMENT_3D('',#37258,#30168,#30169);
#27186=AXIS2_PLACEMENT_3D('',#37264,#30173,#30174);
#27187=AXIS2_PLACEMENT_3D('',#37266,#30175,#30176);
#27188=AXIS2_PLACEMENT_3D('',#37269,#30178,#30179);
#27189=AXIS2_PLACEMENT_3D('',#37270,#30180,#30181);
#27190=AXIS2_PLACEMENT_3D('',#37273,#30183,#30184);
#27191=AXIS2_PLACEMENT_3D('',#37274,#30185,#30186);
#27192=AXIS2_PLACEMENT_3D('',#37276,#30187,#30188);
#27193=AXIS2_PLACEMENT_3D('',#37573,#30190,#30191);
#27194=AXIS2_PLACEMENT_3D('',#37576,#30192,#30193);
#27195=AXIS2_PLACEMENT_3D('',#37577,#30194,#30195);
#27196=AXIS2_PLACEMENT_3D('',#37640,#30199,#30200);
#27197=AXIS2_PLACEMENT_3D('',#37651,#30201,#30202);
#27198=AXIS2_PLACEMENT_3D('',#37654,#30204,#30205);
#27199=AXIS2_PLACEMENT_3D('',#37655,#30206,#30207);
#27200=AXIS2_PLACEMENT_3D('',#37657,#30209,#30210);
#27201=AXIS2_PLACEMENT_3D('',#37666,#30215,#30216);
#27202=AXIS2_PLACEMENT_3D('',#37672,#30220,#30221);
#27203=AXIS2_PLACEMENT_3D('',#37674,#30222,#30223);
#27204=AXIS2_PLACEMENT_3D('',#37677,#30225,#30226);
#27205=AXIS2_PLACEMENT_3D('',#37976,#30230,#30231);
#27206=AXIS2_PLACEMENT_3D('',#37982,#30235,#30236);
#27207=AXIS2_PLACEMENT_3D('',#37988,#30240,#30241);
#27208=AXIS2_PLACEMENT_3D('',#37995,#30245,#30246);
#27209=AXIS2_PLACEMENT_3D('',#38001,#30250,#30251);
#27210=AXIS2_PLACEMENT_3D('',#38008,#30255,#30256);
#27211=AXIS2_PLACEMENT_3D('',#38014,#30260,#30261);
#27212=AXIS2_PLACEMENT_3D('',#38018,#30263,#30264);
#27213=AXIS2_PLACEMENT_3D('',#38019,#30265,#30266);
#27214=AXIS2_PLACEMENT_3D('',#38020,#30267,#30268);
#27215=AXIS2_PLACEMENT_3D('',#38026,#30272,#30273);
#27216=AXIS2_PLACEMENT_3D('',#38030,#30275,#30276);
#27217=AXIS2_PLACEMENT_3D('',#38031,#30277,#30278);
#27218=AXIS2_PLACEMENT_3D('',#38032,#30279,#30280);
#27219=AXIS2_PLACEMENT_3D('',#38035,#30283,#30284);
#27220=AXIS2_PLACEMENT_3D('',#38041,#30288,#30289);
#27221=AXIS2_PLACEMENT_3D('',#38044,#30292,#30293);
#27222=AXIS2_PLACEMENT_3D('',#38047,#30296,#30297);
#27223=AXIS2_PLACEMENT_3D('',#38050,#30300,#30301);
#27224=AXIS2_PLACEMENT_3D('',#38052,#30302,#30303);
#27225=AXIS2_PLACEMENT_3D('',#38054,#30305,#30306);
#27226=AXIS2_PLACEMENT_3D('',#38057,#30308,#30309);
#27227=AXIS2_PLACEMENT_3D('',#38130,#30311,#30312);
#27228=AXIS2_PLACEMENT_3D('',#38136,#30316,#30317);
#27229=AXIS2_PLACEMENT_3D('',#38196,#30319,#30320);
#27230=AXIS2_PLACEMENT_3D('',#38197,#30321,#30322);
#27231=AXIS2_PLACEMENT_3D('',#38208,#30328,#30329);
#27232=AXIS2_PLACEMENT_3D('',#38218,#30334,#30335);
#27233=AXIS2_PLACEMENT_3D('',#38222,#30338,#30339);
#27234=AXIS2_PLACEMENT_3D('',#38223,#30340,#30341);
#27235=AXIS2_PLACEMENT_3D('',#38225,#30343,#30344);
#27236=AXIS2_PLACEMENT_3D('',#38227,#30346,#30347);
#27237=AXIS2_PLACEMENT_3D('',#38228,#30348,#30349);
#27238=AXIS2_PLACEMENT_3D('',#38233,#30351,#30352);
#27239=AXIS2_PLACEMENT_3D('',#38236,#30354,#30355);
#27240=AXIS2_PLACEMENT_3D('',#38241,#30357,#30358);
#27241=AXIS2_PLACEMENT_3D('',#38244,#30360,#30361);
#27242=AXIS2_PLACEMENT_3D('',#38245,#30362,#30363);
#27243=AXIS2_PLACEMENT_3D('',#38251,#30367,#30368);
#27244=AXIS2_PLACEMENT_3D('',#38254,#30370,#30371);
#27245=AXIS2_PLACEMENT_3D('',#38255,#30372,#30373);
#27246=AXIS2_PLACEMENT_3D('',#38259,#30376,#30377);
#27247=AXIS2_PLACEMENT_3D('',#38260,#30378,#30379);
#27248=AXIS2_PLACEMENT_3D('',#38261,#30380,#30381);
#27249=AXIS2_PLACEMENT_3D('',#38265,#30383,#30384);
#27250=AXIS2_PLACEMENT_3D('',#38267,#30386,#30387);
#27251=AXIS2_PLACEMENT_3D('',#38271,#30390,#30391);
#27252=AXIS2_PLACEMENT_3D('',#38277,#30395,#30396);
#27253=AXIS2_PLACEMENT_3D('',#38280,#30398,#30399);
#27254=AXIS2_PLACEMENT_3D('',#38281,#30400,#30401);
#27255=AXIS2_PLACEMENT_3D('',#38285,#30404,#30405);
#27256=AXIS2_PLACEMENT_3D('',#38286,#30406,#30407);
#27257=AXIS2_PLACEMENT_3D('',#38287,#30408,#30409);
#27258=AXIS2_PLACEMENT_3D('',#38291,#30411,#30412);
#27259=AXIS2_PLACEMENT_3D('',#38293,#30414,#30415);
#27260=AXIS2_PLACEMENT_3D('',#38297,#30418,#30419);
#27261=AXIS2_PLACEMENT_3D('',#38303,#30423,#30424);
#27262=AXIS2_PLACEMENT_3D('',#38306,#30426,#30427);
#27263=AXIS2_PLACEMENT_3D('',#38307,#30428,#30429);
#27264=AXIS2_PLACEMENT_3D('',#38311,#30432,#30433);
#27265=AXIS2_PLACEMENT_3D('',#38312,#30434,#30435);
#27266=AXIS2_PLACEMENT_3D('',#38313,#30436,#30437);
#27267=AXIS2_PLACEMENT_3D('',#38317,#30439,#30440);
#27268=AXIS2_PLACEMENT_3D('',#38319,#30442,#30443);
#27269=AXIS2_PLACEMENT_3D('',#38323,#30446,#30447);
#27270=AXIS2_PLACEMENT_3D('',#38329,#30451,#30452);
#27271=AXIS2_PLACEMENT_3D('',#38332,#30454,#30455);
#27272=AXIS2_PLACEMENT_3D('',#38333,#30456,#30457);
#27273=AXIS2_PLACEMENT_3D('',#38337,#30460,#30461);
#27274=AXIS2_PLACEMENT_3D('',#38338,#30462,#30463);
#27275=AXIS2_PLACEMENT_3D('',#38339,#30464,#30465);
#27276=AXIS2_PLACEMENT_3D('',#38343,#30467,#30468);
#27277=AXIS2_PLACEMENT_3D('',#38345,#30470,#30471);
#27278=AXIS2_PLACEMENT_3D('',#38349,#30474,#30475);
#27279=AXIS2_PLACEMENT_3D('',#38351,#30476,#30477);
#27280=AXIS2_PLACEMENT_3D('',#38355,#30479,#30480);
#27281=AXIS2_PLACEMENT_3D('',#38356,#30481,#30482);
#27282=AXIS2_PLACEMENT_3D('',#38357,#30483,#30484);
#27283=AXIS2_PLACEMENT_3D('',#38358,#30485,#30486);
#27284=AXIS2_PLACEMENT_3D('',#38360,#30487,#30488);
#27285=AXIS2_PLACEMENT_3D('',#38362,#30490,#30491);
#27286=AXIS2_PLACEMENT_3D('',#38364,#30492,#30493);
#27287=AXIS2_PLACEMENT_3D('',#38367,#30495,#30496);
#27288=AXIS2_PLACEMENT_3D('',#38368,#30497,#30498);
#27289=AXIS2_PLACEMENT_3D('',#38369,#30499,#30500);
#27290=AXIS2_PLACEMENT_3D('',#38371,#30501,#30502);
#27291=AXIS2_PLACEMENT_3D('',#38373,#30504,#30505);
#27292=AXIS2_PLACEMENT_3D('',#38379,#30509,#30510);
#27293=AXIS2_PLACEMENT_3D('',#38383,#30512,#30513);
#27294=AXIS2_PLACEMENT_3D('',#38384,#30514,#30515);
#27295=AXIS2_PLACEMENT_3D('',#38385,#30516,#30517);
#27296=AXIS2_PLACEMENT_3D('',#38390,#30521,#30522);
#27297=AXIS2_PLACEMENT_3D('',#38391,#30523,#30524);
#27298=AXIS2_PLACEMENT_3D('',#38392,#30525,#30526);
#27299=AXIS2_PLACEMENT_3D('',#38394,#30528,#30529);
#27300=AXIS2_PLACEMENT_3D('',#38428,#30541,#30542);
#27301=AXIS2_PLACEMENT_3D('',#38432,#30544,#30545);
#27302=AXIS2_PLACEMENT_3D('',#38436,#30547,#30548);
#27303=AXIS2_PLACEMENT_3D('',#38439,#30550,#30551);
#27304=AXIS2_PLACEMENT_3D('',#38444,#30553,#30554);
#27305=AXIS2_PLACEMENT_3D('',#38447,#30556,#30557);
#27306=AXIS2_PLACEMENT_3D('',#38452,#30559,#30560);
#27307=AXIS2_PLACEMENT_3D('',#38455,#30562,#30563);
#27308=AXIS2_PLACEMENT_3D('',#38460,#30565,#30566);
#27309=AXIS2_PLACEMENT_3D('',#38463,#30568,#30569);
#27310=AXIS2_PLACEMENT_3D('',#38464,#30570,#30571);
#27311=AXIS2_PLACEMENT_3D('',#38467,#30574,#30575);
#27312=AXIS2_PLACEMENT_3D('',#38470,#30577,#30578);
#27313=AXIS2_PLACEMENT_3D('',#38471,#30579,#30580);
#27314=AXIS2_PLACEMENT_3D('',#38474,#30583,#30584);
#27315=AXIS2_PLACEMENT_3D('',#38475,#30585,#30586);
#27316=AXIS2_PLACEMENT_3D('',#38477,#30588,#30589);
#27317=AXIS2_PLACEMENT_3D('',#38480,#30592,#30593);
#27318=AXIS2_PLACEMENT_3D('',#38483,#30595,#30596);
#27319=AXIS2_PLACEMENT_3D('',#38484,#30597,#30598);
#27320=AXIS2_PLACEMENT_3D('',#38487,#30601,#30602);
#27321=AXIS2_PLACEMENT_3D('',#38488,#30603,#30604);
#27322=AXIS2_PLACEMENT_3D('',#38490,#30606,#30607);
#27323=AXIS2_PLACEMENT_3D('',#38493,#30610,#30611);
#27324=AXIS2_PLACEMENT_3D('',#38496,#30613,#30614);
#27325=AXIS2_PLACEMENT_3D('',#38497,#30615,#30616);
#27326=AXIS2_PLACEMENT_3D('',#38500,#30619,#30620);
#27327=AXIS2_PLACEMENT_3D('',#38501,#30621,#30622);
#27328=AXIS2_PLACEMENT_3D('',#38766,#30625,#30626);
#27329=AXIS2_PLACEMENT_3D('',#38771,#30629,#30630);
#27330=AXIS2_PLACEMENT_3D('',#38772,#30631,#30632);
#27331=AXIS2_PLACEMENT_3D('',#38776,#30635,#30636);
#27332=AXIS2_PLACEMENT_3D('',#38779,#30638,#30639);
#27333=AXIS2_PLACEMENT_3D('',#38780,#30640,#30641);
#27334=AXIS2_PLACEMENT_3D('',#38784,#30644,#30645);
#27335=AXIS2_PLACEMENT_3D('',#38786,#30647,#30648);
#27336=AXIS2_PLACEMENT_3D('',#38787,#30649,#30650);
#27337=AXIS2_PLACEMENT_3D('',#38789,#30652,#30653);
#27338=AXIS2_PLACEMENT_3D('',#38878,#30656,#30657);
#27339=AXIS2_PLACEMENT_3D('',#38879,#30658,#30659);
#27340=AXIS2_PLACEMENT_3D('',#38880,#30660,#30661);
#27341=AXIS2_PLACEMENT_3D('',#38882,#30663,#30664);
#27342=AXIS2_PLACEMENT_3D('',#38884,#30666,#30667);
#27343=AXIS2_PLACEMENT_3D('',#38886,#30669,#30670);
#27344=AXIS2_PLACEMENT_3D('',#38888,#30672,#30673);
#27345=AXIS2_PLACEMENT_3D('',#38897,#30676,#30677);
#27346=AXIS2_PLACEMENT_3D('',#38899,#30678,#30679);
#27347=AXIS2_PLACEMENT_3D('',#38902,#30681,#30682);
#27348=AXIS2_PLACEMENT_3D('',#39077,#30685,#30686);
#27349=AXIS2_PLACEMENT_3D('',#39081,#30689,#30690);
#27350=AXIS2_PLACEMENT_3D('',#39084,#30692,#30693);
#27351=AXIS2_PLACEMENT_3D('',#39085,#30694,#30695);
#27352=AXIS2_PLACEMENT_3D('',#39087,#30697,#30698);
#27353=AXIS2_PLACEMENT_3D('',#39100,#30701,#30702);
#27354=AXIS2_PLACEMENT_3D('',#39143,#30703,#30704);
#27355=AXIS2_PLACEMENT_3D('',#39145,#30706,#30707);
#27356=AXIS2_PLACEMENT_3D('',#39154,#30708,#30709);
#27357=AXIS2_PLACEMENT_3D('',#39155,#30710,#30711);
#27358=AXIS2_PLACEMENT_3D('',#39200,#30713,#30714);
#27359=AXIS2_PLACEMENT_3D('',#39208,#30716,#30717);
#27360=AXIS2_PLACEMENT_3D('',#39209,#30718,#30719);
#27361=AXIS2_PLACEMENT_3D('',#39210,#30720,#30721);
#27362=AXIS2_PLACEMENT_3D('',#39300,#30722,#30723);
#27363=AXIS2_PLACEMENT_3D('',#39311,#30724,#30725);
#27364=AXIS2_PLACEMENT_3D('',#39313,#30727,#30728);
#27365=AXIS2_PLACEMENT_3D('',#39314,#30729,#30730);
#27366=AXIS2_PLACEMENT_3D('',#39315,#30731,#30732);
#27367=AXIS2_PLACEMENT_3D('',#39316,#30733,#30734);
#27368=AXIS2_PLACEMENT_3D('',#39317,#30735,#30736);
#27369=AXIS2_PLACEMENT_3D('',#39318,#30737,#30738);
#27370=AXIS2_PLACEMENT_3D('',#39319,#30739,#30740);
#27371=AXIS2_PLACEMENT_3D('',#39320,#30741,#30742);
#27372=AXIS2_PLACEMENT_3D('',#39321,#30743,#30744);
#27373=AXIS2_PLACEMENT_3D('',#39322,#30745,#30746);
#27374=AXIS2_PLACEMENT_3D('',#39323,#30747,#30748);
#27375=AXIS2_PLACEMENT_3D('',#39324,#30749,#30750);
#27376=AXIS2_PLACEMENT_3D('',#39325,#30751,#30752);
#27377=AXIS2_PLACEMENT_3D('',#39326,#30753,#30754);
#27378=AXIS2_PLACEMENT_3D('',#39327,#30755,#30756);
#27379=AXIS2_PLACEMENT_3D('',#39328,#30757,#30758);
#27380=AXIS2_PLACEMENT_3D('',#39329,#30759,#30760);
#27381=AXIS2_PLACEMENT_3D('',#39332,#30762,#30763);
#27382=AXIS2_PLACEMENT_3D('',#39335,#30765,#30766);
#27383=AXIS2_PLACEMENT_3D('',#39338,#30768,#30769);
#27384=AXIS2_PLACEMENT_3D('',#39341,#30771,#30772);
#27385=AXIS2_PLACEMENT_3D('',#39343,#30773,#30774);
#27386=AXIS2_PLACEMENT_3D('',#39344,#30775,#30776);
#27387=AXIS2_PLACEMENT_3D('',#39384,#30778,#30779);
#27388=AXIS2_PLACEMENT_3D('',#39425,#30781,#30782);
#27389=AXIS2_PLACEMENT_3D('',#39426,#30783,#30784);
#27390=AXIS2_PLACEMENT_3D('',#39428,#30785,#30786);
#27391=AXIS2_PLACEMENT_3D('',#39429,#30787,#30788);
#27392=AXIS2_PLACEMENT_3D('',#39431,#30790,#30791);
#27393=AXIS2_PLACEMENT_3D('',#39433,#30792,#30793);
#27394=AXIS2_PLACEMENT_3D('',#39435,#30795,#30796);
#30055=DIRECTION('axis',(0.,0.,1.));
#30056=DIRECTION('refdir',(1.,0.,0.));
#30057=DIRECTION('center_axis',(0.,-3.00548293115791E-15,-1.));
#30058=DIRECTION('ref_axis',(-1.,-3.13880988628035E-17,0.));
#30059=DIRECTION('center_axis',(0.,0.,-1.));
#30060=DIRECTION('ref_axis',(-1.,0.,0.));
#30061=DIRECTION('',(0.923879532511284,-1.00800709067767E-15,-0.382683432365096));
#30062=DIRECTION('center_axis',(0.,0.,1.));
#30063=DIRECTION('ref_axis',(-1.,-6.12323399573677E-17,0.));
#30064=DIRECTION('center_axis',(0.,0.,1.));
#30065=DIRECTION('ref_axis',(-1.,-6.12323399573677E-17,0.));
#30066=DIRECTION('center_axis',(0.,0.,-1.));
#30067=DIRECTION('ref_axis',(1.,0.,0.));
#30068=DIRECTION('',(-0.707106781186522,-8.65956056235463E-17,-0.707106781186573));
#30069=DIRECTION('center_axis',(0.,0.,-1.));
#30070=DIRECTION('ref_axis',(-1.,-6.12323399573677E-17,0.));
#30071=DIRECTION('center_axis',(0.,0.,-1.));
#30072=DIRECTION('ref_axis',(-1.,-6.12323399573677E-17,0.));
#30073=DIRECTION('center_axis',(0.,0.,1.));
#30074=DIRECTION('ref_axis',(1.,0.,0.));
#30075=DIRECTION('center_axis',(0.,0.,-1.));
#30076=DIRECTION('ref_axis',(1.,0.,0.));
#30077=DIRECTION('center_axis',(0.,1.26592340881653E-15,-1.));
#30078=DIRECTION('ref_axis',(-1.,-3.0312508555666E-17,0.));
#30079=DIRECTION('',(0.382683432365077,1.22802602600346E-15,-0.923879532511292));
#30080=DIRECTION('center_axis',(0.,0.,1.));
#30081=DIRECTION('ref_axis',(-1.,0.,0.));
#30082=DIRECTION('center_axis',(0.,0.,1.));
#30083=DIRECTION('ref_axis',(-1.,0.,0.));
#30084=DIRECTION('center_axis',(0.,0.,1.));
#30085=DIRECTION('ref_axis',(1.,0.,0.));
#30086=DIRECTION('',(0.,0.,-1.));
#30087=DIRECTION('center_axis',(-1.,0.,0.));
#30088=DIRECTION('ref_axis',(0.,0.,-1.));
#30089=DIRECTION('center_axis',(-1.,0.,0.));
#30090=DIRECTION('ref_axis',(0.,0.,-1.));
#30091=DIRECTION('',(0.707106781186538,-8.65956056235505E-17,-0.707106781186557));
#30092=DIRECTION('center_axis',(1.,0.,0.));
#30093=DIRECTION('ref_axis',(0.,0.,-1.));
#30094=DIRECTION('center_axis',(1.,0.,0.));
#30095=DIRECTION('ref_axis',(0.,0.,-1.));
#30096=DIRECTION('center_axis',(-1.,0.,0.));
#30097=DIRECTION('ref_axis',(0.,0.,-1.));
#30098=DIRECTION('center_axis',(1.,0.,0.));
#30099=DIRECTION('ref_axis',(0.,-1.,0.));
#30100=DIRECTION('center_axis',(-1.,0.,0.));
#30101=DIRECTION('ref_axis',(0.,-1.,0.));
#30102=DIRECTION('center_axis',(-1.,0.,0.));
#30103=DIRECTION('ref_axis',(0.,-1.,0.));
#30104=DIRECTION('',(-0.707106781186546,-0.707106781186549,-8.65956056235495E-17));
#30105=DIRECTION('center_axis',(1.,0.,0.));
#30106=DIRECTION('ref_axis',(0.,-1.,0.));
#30107=DIRECTION('center_axis',(1.,0.,0.));
#30108=DIRECTION('ref_axis',(0.,-1.,0.));
#30109=DIRECTION('center_axis',(1.,0.,0.));
#30110=DIRECTION('ref_axis',(0.,-1.,0.));
#30111=DIRECTION('center_axis',(1.,0.,0.));
#30112=DIRECTION('ref_axis',(0.,-1.,0.));
#30113=DIRECTION('center_axis',(1.,0.,0.));
#30114=DIRECTION('ref_axis',(0.,-1.,0.));
#30115=DIRECTION('center_axis',(-1.,0.,0.));
#30116=DIRECTION('ref_axis',(0.,0.,1.));
#30117=DIRECTION('center_axis',(-1.,0.,0.));
#30118=DIRECTION('ref_axis',(0.,0.,1.));
#30119=DIRECTION('',(-1.,0.,0.));
#30120=DIRECTION('center_axis',(-1.,0.,0.));
#30121=DIRECTION('ref_axis',(0.,0.,1.));
#30122=DIRECTION('center_axis',(-1.,0.,0.));
#30123=DIRECTION('ref_axis',(0.,0.,1.));
#30124=DIRECTION('',(0.707106781186562,8.65956056235476E-17,0.707106781186533));
#30125=DIRECTION('center_axis',(1.,0.,0.));
#30126=DIRECTION('ref_axis',(0.,0.,1.));
#30127=DIRECTION('center_axis',(-1.,0.,0.));
#30128=DIRECTION('ref_axis',(0.,0.,1.));
#30129=DIRECTION('center_axis',(-1.,0.,0.));
#30130=DIRECTION('ref_axis',(0.,0.,1.));
#30131=DIRECTION('center_axis',(-1.,0.,0.));
#30132=DIRECTION('ref_axis',(0.,0.,1.));
#30133=DIRECTION('',(-1.,0.,0.));
#30134=DIRECTION('center_axis',(-0.707106781186541,0.,-0.707106781186554));
#30135=DIRECTION('ref_axis',(-0.707106781186554,0.,0.707106781186541));
#30136=DIRECTION('',(0.577350269189629,-0.577350269189629,-0.577350269189619));
#30137=DIRECTION('',(0.,-1.,0.));
#30138=DIRECTION('',(-0.577350269189629,-0.577350269189629,0.577350269189619));
#30139=DIRECTION('',(-0.577350269189629,0.577350269189629,0.577350269189619));
#30140=DIRECTION('',(0.,1.,0.));
#30141=DIRECTION('',(0.577350269189629,0.577350269189629,-0.577350269189619));
#30142=DIRECTION('center_axis',(0.,0.,1.));
#30143=DIRECTION('ref_axis',(1.,0.,0.));
#30144=DIRECTION('',(-1.,0.,0.));
#30145=DIRECTION('center_axis',(0.,0.,1.));
#30146=DIRECTION('ref_axis',(1.,1.77635683940025E-15,0.));
#30147=DIRECTION('',(0.,1.,0.));
#30148=DIRECTION('center_axis',(0.,0.,1.));
#30149=DIRECTION('ref_axis',(0.,-1.,0.));
#30150=DIRECTION('',(1.,0.,0.));
#30151=DIRECTION('',(0.,1.,0.));
#30152=DIRECTION('center_axis',(0.,0.,-1.));
#30153=DIRECTION('ref_axis',(-1.,3.22973970800045E-15,0.));
#30154=DIRECTION('',(0.,-1.,0.));
#30155=DIRECTION('center_axis',(0.,0.,-1.));
#30156=DIRECTION('ref_axis',(1.,-3.22973970800045E-15,0.));
#30157=DIRECTION('',(0.,1.,0.));
#30158=DIRECTION('center_axis',(0.,0.,-1.));
#30159=DIRECTION('ref_axis',(-1.,3.22973970800045E-15,0.));
#30160=DIRECTION('',(0.,-1.,0.));
#30161=DIRECTION('center_axis',(0.,0.,-1.));
#30162=DIRECTION('ref_axis',(1.,-3.22973970800045E-15,0.));
#30163=DIRECTION('center_axis',(0.,0.707106781186541,-0.707106781186554));
#30164=DIRECTION('ref_axis',(-1.,0.,0.));
#30165=DIRECTION('',(-0.577350269189629,-0.577350269189629,-0.577350269189619));
#30166=DIRECTION('',(1.,0.,0.));
#30167=DIRECTION('',(0.,-0.707106781186554,-0.707106781186541));
#30168=DIRECTION('center_axis',(-0.707106781186548,0.707106781186548,0.));
#30169=DIRECTION('ref_axis',(0.,0.,1.));
#30170=DIRECTION('',(0.,0.,1.));
#30171=DIRECTION('',(0.577350269189622,0.577350269189643,0.577350269189612));
#30172=DIRECTION('',(0.,0.,-1.));
#30173=DIRECTION('center_axis',(-1.,0.,0.));
#30174=DIRECTION('ref_axis',(0.,-1.,0.));
#30175=DIRECTION('center_axis',(1.,0.,0.));
#30176=DIRECTION('ref_axis',(0.,-1.,0.));
#30177=DIRECTION('',(0.382683432365096,-0.923879532511284,1.1314261122877E-16));
#30178=DIRECTION('center_axis',(-1.,0.,0.));
#30179=DIRECTION('ref_axis',(0.,-1.,0.));
#30180=DIRECTION('center_axis',(-1.,0.,0.));
#30181=DIRECTION('ref_axis',(0.,-1.,0.));
#30182=DIRECTION('',(-0.707106781186552,0.707106781186543,8.65956056235488E-17));
#30183=DIRECTION('center_axis',(-1.,0.,0.));
#30184=DIRECTION('ref_axis',(0.,-1.,0.));
#30185=DIRECTION('center_axis',(1.,0.,0.));
#30186=DIRECTION('ref_axis',(0.,0.,-1.));
#30187=DIRECTION('center_axis',(-1.,0.,0.));
#30188=DIRECTION('ref_axis',(0.,1.,0.));
#30189=DIRECTION('',(0.,0.75225657268058,0.658870282270242));
#30190=DIRECTION('center_axis',(1.,0.,0.));
#30191=DIRECTION('ref_axis',(0.,1.,0.));
#30192=DIRECTION('center_axis',(1.,0.,0.));
#30193=DIRECTION('ref_axis',(0.,-1.,0.));
#30194=DIRECTION('center_axis',(1.,0.,0.));
#30195=DIRECTION('ref_axis',(0.,-1.,0.));
#30196=DIRECTION('',(-1.,0.,0.));
#30197=DIRECTION('',(-1.,0.,0.));
#30198=DIRECTION('',(1.,0.,0.));
#30199=DIRECTION('center_axis',(-1.,0.,0.));
#30200=DIRECTION('ref_axis',(0.,2.83276944882399E-16,-1.));
#30201=DIRECTION('center_axis',(0.,0.,1.));
#30202=DIRECTION('ref_axis',(1.,0.,0.));
#30203=DIRECTION('',(0.,0.,1.));
#30204=DIRECTION('center_axis',(0.,0.,1.));
#30205=DIRECTION('ref_axis',(1.,0.,0.));
#30206=DIRECTION('center_axis',(-1.,0.,0.));
#30207=DIRECTION('ref_axis',(0.,-1.,0.));
#30208=DIRECTION('',(-0.923879532511285,0.382683432365094,4.68652040532634E-17));
#30209=DIRECTION('center_axis',(-0.707106781186541,-0.707106781186554,0.));
#30210=DIRECTION('ref_axis',(0.,0.,1.));
#30211=DIRECTION('',(-0.706643908451704,0.706643908451754,0.0361769719037954));
#30212=DIRECTION('',(0.,0.,-1.));
#30213=DIRECTION('',(-0.707106781186554,0.707106781186541,0.));
#30214=DIRECTION('',(0.,0.,1.));
#30215=DIRECTION('center_axis',(1.,0.,0.));
#30216=DIRECTION('ref_axis',(0.,0.,-1.));
#30217=DIRECTION('',(0.,1.,0.));
#30218=DIRECTION('',(0.,-0.256212647338981,0.966620442233429));
#30219=DIRECTION('',(0.,-1.,0.));
#30220=DIRECTION('center_axis',(0.,1.,0.));
#30221=DIRECTION('ref_axis',(-0.999937018558663,0.,0.0112231419848006));
#30222=DIRECTION('center_axis',(0.,1.,0.));
#30223=DIRECTION('ref_axis',(-0.999937018558664,0.,0.0112231419848006));
#30224=DIRECTION('',(-0.659148681788774,0.707106781186549,0.255974637993922));
#30225=DIRECTION('center_axis',(0.,-1.,0.));
#30226=DIRECTION('ref_axis',(-0.999937018558664,0.,0.0112231419848006));
#30227=DIRECTION('',(-2.99369449574795E-14,-0.877058019307039,0.480384461415243));
#30228=DIRECTION('',(2.99369449574799E-14,-0.877058019307036,-0.480384461415249));
#30229=DIRECTION('',(0.468387297258231,0.511424326802648,0.720457144958386));
#30230=DIRECTION('center_axis',(0.,-0.707106781186541,-0.707106781186554));
#30231=DIRECTION('ref_axis',(-1.,0.,0.));
#30232=DIRECTION('',(0.,-0.707106781186554,0.707106781186541));
#30233=DIRECTION('',(-1.,0.,0.));
#30234=DIRECTION('',(-0.577350269189629,0.577350269189629,-0.577350269189619));
#30235=DIRECTION('center_axis',(-0.707106781186548,-0.707106781186548,0.));
#30236=DIRECTION('ref_axis',(0.,0.,1.));
#30237=DIRECTION('',(0.,0.,1.));
#30238=DIRECTION('',(-0.577350269189629,0.577350269189629,-0.577350269189619));
#30239=DIRECTION('',(0.,0.,-1.));
#30240=DIRECTION('center_axis',(0.577350269189622,-0.577350269189622,-0.577350269189633));
#30241=DIRECTION('ref_axis',(-0.707106781186554,0.,-0.707106781186541));
#30242=DIRECTION('',(-0.707106781186554,0.,-0.707106781186541));
#30243=DIRECTION('',(0.707106781186548,0.707106781186548,0.));
#30244=DIRECTION('',(0.,-0.707106781186554,0.707106781186541));
#30245=DIRECTION('center_axis',(0.707106781186548,-0.707106781186548,0.));
#30246=DIRECTION('ref_axis',(0.,0.,-1.));
#30247=DIRECTION('',(0.,0.,-1.));
#30248=DIRECTION('',(0.,0.,1.));
#30249=DIRECTION('',(-0.577350269189622,-0.577350269189643,0.577350269189612));
#30250=DIRECTION('center_axis',(0.577350269189622,0.577350269189622,-0.577350269189633));
#30251=DIRECTION('ref_axis',(-0.707106781186554,0.,-0.707106781186541));
#30252=DIRECTION('',(0.707106781186554,0.,0.707106781186541));
#30253=DIRECTION('',(0.,-0.707106781186554,-0.707106781186541));
#30254=DIRECTION('',(-0.707106781186548,0.707106781186548,0.));
#30255=DIRECTION('center_axis',(0.,0.707106781186541,-0.707106781186554));
#30256=DIRECTION('ref_axis',(-1.,0.,0.));
#30257=DIRECTION('',(0.,0.707106781186554,0.707106781186541));
#30258=DIRECTION('',(1.,0.,0.));
#30259=DIRECTION('',(-1.,0.,0.));
#30260=DIRECTION('center_axis',(0.,0.,1.));
#30261=DIRECTION('ref_axis',(0.,1.,0.));
#30262=DIRECTION('',(-0.707106781186554,0.,0.707106781186541));
#30263=DIRECTION('center_axis',(0.,0.,-1.));
#30264=DIRECTION('ref_axis',(0.,1.,0.));
#30265=DIRECTION('center_axis',(0.,0.,1.));
#30266=DIRECTION('ref_axis',(0.,1.,0.));
#30267=DIRECTION('center_axis',(-0.707106781186541,0.,-0.707106781186554));
#30268=DIRECTION('ref_axis',(-0.707106781186554,0.,0.707106781186541));
#30269=DIRECTION('',(-0.707106781186554,0.,0.707106781186541));
#30270=DIRECTION('',(0.,1.,0.));
#30271=DIRECTION('',(0.,-1.,0.));
#30272=DIRECTION('center_axis',(0.,0.,1.));
#30273=DIRECTION('ref_axis',(-1.,0.,0.));
#30274=DIRECTION('',(0.,-0.707106781186554,0.707106781186541));
#30275=DIRECTION('center_axis',(0.,0.,-1.));
#30276=DIRECTION('ref_axis',(-1.,0.,0.));
#30277=DIRECTION('center_axis',(0.,0.,1.));
#30278=DIRECTION('ref_axis',(-1.,0.,0.));
#30279=DIRECTION('center_axis',(0.,-0.707106781186541,-0.707106781186554));
#30280=DIRECTION('ref_axis',(-1.,0.,0.));
#30281=DIRECTION('',(1.,0.,0.));
#30282=DIRECTION('',(-1.,0.,0.));
#30283=DIRECTION('center_axis',(0.707106781186548,0.707106781186548,0.));
#30284=DIRECTION('ref_axis',(0.,0.,-1.));
#30285=DIRECTION('',(0.,0.,-1.));
#30286=DIRECTION('',(0.,0.,1.));
#30287=DIRECTION('',(0.577350269189629,-0.577350269189629,-0.577350269189619));
#30288=DIRECTION('center_axis',(0.707106781186541,0.,-0.707106781186554));
#30289=DIRECTION('ref_axis',(-0.707106781186554,0.,-0.707106781186541));
#30290=DIRECTION('',(0.,1.,0.));
#30291=DIRECTION('',(0.,-1.,0.));
#30292=DIRECTION('center_axis',(0.,0.707106781186541,-0.707106781186554));
#30293=DIRECTION('ref_axis',(-1.,0.,0.));
#30294=DIRECTION('',(-1.,0.,0.));
#30295=DIRECTION('',(1.,0.,0.));
#30296=DIRECTION('center_axis',(0.,-0.707106781186541,-0.707106781186554));
#30297=DIRECTION('ref_axis',(-1.,0.,0.));
#30298=DIRECTION('',(-1.,0.,0.));
#30299=DIRECTION('',(1.,0.,0.));
#30300=DIRECTION('center_axis',(0.,0.,1.));
#30301=DIRECTION('ref_axis',(1.,1.77635683940025E-15,0.));
#30302=DIRECTION('center_axis',(0.,0.,-1.));
#30303=DIRECTION('ref_axis',(1.,1.77635683940025E-15,0.));
#30304=DIRECTION('',(-0.49497474683058,-0.50497524691812,-0.707106781186538));
#30305=DIRECTION('center_axis',(0.,0.,1.));
#30306=DIRECTION('ref_axis',(0.,-1.,0.));
#30307=DIRECTION('',(0.494974746830587,-0.504975246918101,0.707106781186547));
#30308=DIRECTION('center_axis',(0.,0.,-1.));
#30309=DIRECTION('ref_axis',(0.,-1.,0.));
#30310=DIRECTION('',(-0.468387297258238,0.511424326802607,-0.72045714495841));
#30311=DIRECTION('center_axis',(0.,-1.,0.));
#30312=DIRECTION('ref_axis',(1.,0.,0.));
#30313=DIRECTION('',(0.,0.,1.));
#30314=DIRECTION('',(1.,0.,0.));
#30315=DIRECTION('',(0.,0.,1.));
#30316=DIRECTION('center_axis',(0.,0.,1.));
#30317=DIRECTION('ref_axis',(0.,-1.,0.));
#30318=DIRECTION('',(0.,0.,1.));
#30319=DIRECTION('center_axis',(0.,0.,1.));
#30320=DIRECTION('ref_axis',(0.,-1.,0.));
#30321=DIRECTION('center_axis',(1.,0.,0.));
#30322=DIRECTION('ref_axis',(0.,0.,-1.));
#30323=DIRECTION('',(0.,-1.,0.));
#30324=DIRECTION('',(0.,0.,1.));
#30325=DIRECTION('',(0.,0.877058019307042,-0.480384461415237));
#30326=DIRECTION('',(0.,1.,0.));
#30327=DIRECTION('',(0.,0.256212647338981,-0.966620442233429));
#30328=DIRECTION('center_axis',(1.,0.,0.));
#30329=DIRECTION('ref_axis',(0.,2.83276944882399E-16,-1.));
#30330=DIRECTION('',(0.,0.256212647338981,0.966620442233429));
#30331=DIRECTION('',(0.,1.,0.));
#30332=DIRECTION('',(0.,0.877058019307039,0.480384461415243));
#30333=DIRECTION('',(0.,0.,-1.));
#30334=DIRECTION('center_axis',(1.,0.,0.));
#30335=DIRECTION('ref_axis',(0.,6.12323399573677E-17,1.));
#30336=DIRECTION('',(0.,0.,1.));
#30337=DIRECTION('',(0.,1.,0.));
#30338=DIRECTION('center_axis',(0.,1.,0.));
#30339=DIRECTION('ref_axis',(0.707106781186543,0.,-0.707106781186552));
#30340=DIRECTION('center_axis',(-1.,0.,0.));
#30341=DIRECTION('ref_axis',(0.,-1.,0.));
#30342=DIRECTION('',(0.,-1.,0.));
#30343=DIRECTION('center_axis',(1.,0.,0.));
#30344=DIRECTION('ref_axis',(0.,1.,0.));
#30345=DIRECTION('',(0.,1.,0.));
#30346=DIRECTION('center_axis',(0.,0.,1.));
#30347=DIRECTION('ref_axis',(1.,0.,0.));
#30348=DIRECTION('center_axis',(0.,0.,1.));
#30349=DIRECTION('ref_axis',(1.,0.,0.));
#30350=DIRECTION('',(0.,1.,0.));
#30351=DIRECTION('center_axis',(0.,0.,-1.));
#30352=DIRECTION('ref_axis',(-1.,0.,0.));
#30353=DIRECTION('',(0.,-1.,0.));
#30354=DIRECTION('center_axis',(0.,0.,-1.));
#30355=DIRECTION('ref_axis',(1.,0.,0.));
#30356=DIRECTION('',(0.,1.,0.));
#30357=DIRECTION('center_axis',(0.,0.,-1.));
#30358=DIRECTION('ref_axis',(-1.,0.,0.));
#30359=DIRECTION('',(0.,-1.,0.));
#30360=DIRECTION('center_axis',(0.,0.,-1.));
#30361=DIRECTION('ref_axis',(1.,0.,0.));
#30362=DIRECTION('center_axis',(0.707106781186566,0.,-0.707106781186529));
#30363=DIRECTION('ref_axis',(-0.707106781186529,0.,-0.707106781186566));
#30364=DIRECTION('',(-0.707106781186529,0.,-0.707106781186566));
#30365=DIRECTION('',(0.707106781186529,0.,0.707106781186566));
#30366=DIRECTION('',(0.,-1.,0.));
#30367=DIRECTION('center_axis',(0.,0.,-1.));
#30368=DIRECTION('ref_axis',(-1.,3.22973970800045E-15,0.));
#30369=DIRECTION('',(0.707106781186554,0.,-0.707106781186541));
#30370=DIRECTION('center_axis',(0.,0.,1.));
#30371=DIRECTION('ref_axis',(-1.,3.22973970800045E-15,0.));
#30372=DIRECTION('center_axis',(-0.707106781186566,0.,-0.707106781186529));
#30373=DIRECTION('ref_axis',(-0.707106781186529,0.,0.707106781186566));
#30374=DIRECTION('',(0.707106781186529,0.,-0.707106781186566));
#30375=DIRECTION('',(0.,1.,0.));
#30376=DIRECTION('center_axis',(0.,0.,-1.));
#30377=DIRECTION('ref_axis',(1.,-3.22973970800045E-15,0.));
#30378=DIRECTION('center_axis',(0.,0.,1.));
#30379=DIRECTION('ref_axis',(1.,-3.22973970800045E-15,0.));
#30380=DIRECTION('center_axis',(0.,0.,-1.));
#30381=DIRECTION('ref_axis',(-1.,3.22973970800045E-15,0.));
#30382=DIRECTION('',(0.,0.,-1.));
#30383=DIRECTION('center_axis',(0.,0.,-1.));
#30384=DIRECTION('ref_axis',(-1.,3.22973970800045E-15,0.));
#30385=DIRECTION('',(0.,0.,-1.));
#30386=DIRECTION('center_axis',(-1.,0.,0.));
#30387=DIRECTION('ref_axis',(0.,1.,0.));
#30388=DIRECTION('',(0.,0.,-1.));
#30389=DIRECTION('',(0.,1.,0.));
#30390=DIRECTION('center_axis',(0.707106781186541,0.,-0.707106781186554));
#30391=DIRECTION('ref_axis',(-0.707106781186554,0.,-0.707106781186541));
#30392=DIRECTION('',(-0.707106781186554,0.,-0.707106781186541));
#30393=DIRECTION('',(0.707106781186554,0.,0.707106781186541));
#30394=DIRECTION('',(0.,-1.,0.));
#30395=DIRECTION('center_axis',(0.,0.,-1.));
#30396=DIRECTION('ref_axis',(-1.,0.,0.));
#30397=DIRECTION('',(0.707106781186554,0.,-0.707106781186541));
#30398=DIRECTION('center_axis',(0.,0.,1.));
#30399=DIRECTION('ref_axis',(-1.,0.,0.));
#30400=DIRECTION('center_axis',(-0.707106781186541,0.,-0.707106781186554));
#30401=DIRECTION('ref_axis',(-0.707106781186554,0.,0.707106781186541));
#30402=DIRECTION('',(0.707106781186554,0.,-0.707106781186541));
#30403=DIRECTION('',(0.,1.,0.));
#30404=DIRECTION('center_axis',(0.,0.,-1.));
#30405=DIRECTION('ref_axis',(1.,0.,0.));
#30406=DIRECTION('center_axis',(0.,0.,1.));
#30407=DIRECTION('ref_axis',(1.,0.,0.));
#30408=DIRECTION('center_axis',(0.,0.,-1.));
#30409=DIRECTION('ref_axis',(-1.,0.,0.));
#30410=DIRECTION('',(0.,0.,-1.));
#30411=DIRECTION('center_axis',(0.,0.,-1.));
#30412=DIRECTION('ref_axis',(-1.,0.,0.));
#30413=DIRECTION('',(0.,0.,-1.));
#30414=DIRECTION('center_axis',(-1.,0.,0.));
#30415=DIRECTION('ref_axis',(0.,1.,0.));
#30416=DIRECTION('',(0.,0.,-1.));
#30417=DIRECTION('',(0.,1.,0.));
#30418=DIRECTION('center_axis',(0.707106781186541,0.,-0.707106781186554));
#30419=DIRECTION('ref_axis',(-0.707106781186554,0.,-0.707106781186541));
#30420=DIRECTION('',(-0.707106781186554,0.,-0.707106781186541));
#30421=DIRECTION('',(0.707106781186554,0.,0.707106781186541));
#30422=DIRECTION('',(0.,-1.,0.));
#30423=DIRECTION('center_axis',(0.,0.,-1.));
#30424=DIRECTION('ref_axis',(-1.,0.,0.));
#30425=DIRECTION('',(0.707106781186554,0.,-0.707106781186541));
#30426=DIRECTION('center_axis',(0.,0.,1.));
#30427=DIRECTION('ref_axis',(-1.,0.,0.));
#30428=DIRECTION('center_axis',(-0.707106781186541,0.,-0.707106781186554));
#30429=DIRECTION('ref_axis',(-0.707106781186554,0.,0.707106781186541));
#30430=DIRECTION('',(0.707106781186554,0.,-0.707106781186541));
#30431=DIRECTION('',(0.,1.,0.));
#30432=DIRECTION('center_axis',(0.,0.,-1.));
#30433=DIRECTION('ref_axis',(1.,0.,0.));
#30434=DIRECTION('center_axis',(0.,0.,1.));
#30435=DIRECTION('ref_axis',(1.,0.,0.));
#30436=DIRECTION('center_axis',(0.,0.,-1.));
#30437=DIRECTION('ref_axis',(-1.,0.,0.));
#30438=DIRECTION('',(0.,0.,-1.));
#30439=DIRECTION('center_axis',(0.,0.,-1.));
#30440=DIRECTION('ref_axis',(-1.,0.,0.));
#30441=DIRECTION('',(0.,0.,-1.));
#30442=DIRECTION('center_axis',(-1.,0.,0.));
#30443=DIRECTION('ref_axis',(0.,1.,0.));
#30444=DIRECTION('',(0.,0.,-1.));
#30445=DIRECTION('',(0.,1.,0.));
#30446=DIRECTION('center_axis',(0.707106781186566,0.,-0.707106781186529));
#30447=DIRECTION('ref_axis',(-0.707106781186529,0.,-0.707106781186566));
#30448=DIRECTION('',(-0.707106781186529,0.,-0.707106781186566));
#30449=DIRECTION('',(0.707106781186529,0.,0.707106781186566));
#30450=DIRECTION('',(0.,-1.,0.));
#30451=DIRECTION('center_axis',(0.,0.,-1.));
#30452=DIRECTION('ref_axis',(-1.,3.22973970800045E-15,0.));
#30453=DIRECTION('',(0.707106781186554,0.,-0.707106781186541));
#30454=DIRECTION('center_axis',(0.,0.,1.));
#30455=DIRECTION('ref_axis',(-1.,3.22973970800045E-15,0.));
#30456=DIRECTION('center_axis',(-0.707106781186566,0.,-0.707106781186529));
#30457=DIRECTION('ref_axis',(-0.707106781186529,0.,0.707106781186566));
#30458=DIRECTION('',(0.707106781186529,0.,-0.707106781186566));
#30459=DIRECTION('',(0.,1.,0.));
#30460=DIRECTION('center_axis',(0.,0.,-1.));
#30461=DIRECTION('ref_axis',(1.,-3.22973970800045E-15,0.));
#30462=DIRECTION('center_axis',(0.,0.,1.));
#30463=DIRECTION('ref_axis',(1.,-3.22973970800045E-15,0.));
#30464=DIRECTION('center_axis',(0.,0.,-1.));
#30465=DIRECTION('ref_axis',(-1.,3.22973970800045E-15,0.));
#30466=DIRECTION('',(0.,0.,-1.));
#30467=DIRECTION('center_axis',(0.,0.,-1.));
#30468=DIRECTION('ref_axis',(-1.,3.22973970800045E-15,0.));
#30469=DIRECTION('',(0.,0.,-1.));
#30470=DIRECTION('center_axis',(-1.,0.,0.));
#30471=DIRECTION('ref_axis',(0.,1.,0.));
#30472=DIRECTION('',(0.,0.,-1.));
#30473=DIRECTION('',(0.,1.,0.));
#30474=DIRECTION('center_axis',(-1.,0.,0.));
#30475=DIRECTION('ref_axis',(0.,0.,-1.));
#30476=DIRECTION('center_axis',(-1.,0.,0.));
#30477=DIRECTION('ref_axis',(0.,0.,-1.));
#30478=DIRECTION('',(0.707106781186538,-8.65956056235505E-17,-0.707106781186557));
#30479=DIRECTION('center_axis',(1.,0.,0.));
#30480=DIRECTION('ref_axis',(0.,0.,-1.));
#30481=DIRECTION('center_axis',(1.,0.,0.));
#30482=DIRECTION('ref_axis',(0.,0.,-1.));
#30483=DIRECTION('center_axis',(-1.,0.,0.));
#30484=DIRECTION('ref_axis',(0.,0.,-1.));
#30485=DIRECTION('center_axis',(-1.,0.,0.));
#30486=DIRECTION('ref_axis',(0.,0.,1.));
#30487=DIRECTION('center_axis',(-1.,0.,0.));
#30488=DIRECTION('ref_axis',(0.,0.,1.));
#30489=DIRECTION('',(-1.,0.,0.));
#30490=DIRECTION('center_axis',(-1.,0.,0.));
#30491=DIRECTION('ref_axis',(0.,0.,1.));
#30492=DIRECTION('center_axis',(-1.,0.,0.));
#30493=DIRECTION('ref_axis',(0.,0.,1.));
#30494=DIRECTION('',(0.707106781186542,8.659560562355E-17,0.707106781186553));
#30495=DIRECTION('center_axis',(1.,0.,0.));
#30496=DIRECTION('ref_axis',(0.,0.,1.));
#30497=DIRECTION('center_axis',(-1.,0.,0.));
#30498=DIRECTION('ref_axis',(0.,0.,1.));
#30499=DIRECTION('center_axis',(-1.,0.,0.));
#30500=DIRECTION('ref_axis',(0.,0.,1.));
#30501=DIRECTION('center_axis',(-1.,0.,0.));
#30502=DIRECTION('ref_axis',(0.,0.,1.));
#30503=DIRECTION('',(-1.,0.,0.));
#30504=DIRECTION('center_axis',(0.707106781186566,0.,0.707106781186529));
#30505=DIRECTION('ref_axis',(0.707106781186529,0.,-0.707106781186566));
#30506=DIRECTION('',(-0.707106781186529,0.,0.707106781186566));
#30507=DIRECTION('',(0.,-1.,0.));
#30508=DIRECTION('',(0.707106781186529,0.,-0.707106781186566));
#30509=DIRECTION('center_axis',(0.,0.,1.));
#30510=DIRECTION('ref_axis',(1.,-3.22973970800045E-15,0.));
#30511=DIRECTION('',(0.707106781186554,0.,0.707106781186541));
#30512=DIRECTION('center_axis',(0.,0.,1.));
#30513=DIRECTION('ref_axis',(1.,-3.22973970800045E-15,0.));
#30514=DIRECTION('center_axis',(0.,0.,-1.));
#30515=DIRECTION('ref_axis',(1.,-3.22973970800045E-15,0.));
#30516=DIRECTION('center_axis',(-0.707106781186566,0.,0.707106781186529));
#30517=DIRECTION('ref_axis',(0.707106781186529,0.,0.707106781186566));
#30518=DIRECTION('',(0.707106781186529,0.,0.707106781186566));
#30519=DIRECTION('',(0.,1.,0.));
#30520=DIRECTION('',(0.,-1.,0.));
#30521=DIRECTION('center_axis',(0.,0.,1.));
#30522=DIRECTION('ref_axis',(-1.,3.22973970800045E-15,0.));
#30523=DIRECTION('center_axis',(0.,0.,1.));
#30524=DIRECTION('ref_axis',(-1.,3.22973970800045E-15,0.));
#30525=DIRECTION('center_axis',(0.,0.,-1.));
#30526=DIRECTION('ref_axis',(1.,-3.22973970800045E-15,0.));
#30527=DIRECTION('',(0.,0.,-1.));
#30528=DIRECTION('center_axis',(0.,0.,1.));
#30529=DIRECTION('ref_axis',(1.,0.,0.));
#30530=DIRECTION('',(0.,-1.,0.));
#30531=DIRECTION('',(1.,0.,0.));
#30532=DIRECTION('',(-0.695004915696666,0.719004984097795,0.));
#30533=DIRECTION('',(0.,-1.,0.));
#30534=DIRECTION('',(0.707106781186554,0.707106781186541,0.));
#30535=DIRECTION('',(1.,0.,0.));
#30536=DIRECTION('',(0.,-1.,0.));
#30537=DIRECTION('',(1.,0.,0.));
#30538=DIRECTION('',(0.69500491569666,0.719004984097801,0.));
#30539=DIRECTION('',(1.,0.,0.));
#30540=DIRECTION('',(0.,-1.,0.));
#30541=DIRECTION('center_axis',(0.,0.,-1.));
#30542=DIRECTION('ref_axis',(1.,1.77635683940025E-15,0.));
#30543=DIRECTION('',(1.,0.,0.));
#30544=DIRECTION('center_axis',(0.,0.,-1.));
#30545=DIRECTION('ref_axis',(0.,1.,0.));
#30546=DIRECTION('',(0.,1.,0.));
#30547=DIRECTION('center_axis',(0.,0.,-1.));
#30548=DIRECTION('ref_axis',(-1.,0.,0.));
#30549=DIRECTION('',(-1.,0.,0.));
#30550=DIRECTION('center_axis',(0.,0.,-1.));
#30551=DIRECTION('ref_axis',(0.,-1.,0.));
#30552=DIRECTION('',(0.,-1.,0.));
#30553=DIRECTION('center_axis',(0.,0.,1.));
#30554=DIRECTION('ref_axis',(1.,0.,0.));
#30555=DIRECTION('',(0.,1.,0.));
#30556=DIRECTION('center_axis',(0.,0.,1.));
#30557=DIRECTION('ref_axis',(-1.,0.,0.));
#30558=DIRECTION('',(0.,-1.,0.));
#30559=DIRECTION('center_axis',(0.,0.,1.));
#30560=DIRECTION('ref_axis',(1.,-3.22973970800045E-15,0.));
#30561=DIRECTION('',(0.,1.,0.));
#30562=DIRECTION('center_axis',(0.,0.,1.));
#30563=DIRECTION('ref_axis',(-1.,3.22973970800045E-15,0.));
#30564=DIRECTION('',(0.,-1.,0.));
#30565=DIRECTION('center_axis',(0.,0.,1.));
#30566=DIRECTION('ref_axis',(1.,0.,0.));
#30567=DIRECTION('',(0.,1.,0.));
#30568=DIRECTION('center_axis',(0.,0.,1.));
#30569=DIRECTION('ref_axis',(-1.,0.,0.));
#30570=DIRECTION('center_axis',(0.707106781186541,0.,0.707106781186554));
#30571=DIRECTION('ref_axis',(0.707106781186554,0.,-0.707106781186541));
#30572=DIRECTION('',(-0.707106781186554,0.,0.707106781186541));
#30573=DIRECTION('',(0.707106781186554,0.,-0.707106781186541));
#30574=DIRECTION('center_axis',(0.,0.,1.));
#30575=DIRECTION('ref_axis',(1.,0.,0.));
#30576=DIRECTION('',(0.707106781186554,0.,0.707106781186541));
#30577=DIRECTION('center_axis',(0.,0.,-1.));
#30578=DIRECTION('ref_axis',(1.,0.,0.));
#30579=DIRECTION('center_axis',(-0.707106781186541,0.,0.707106781186554));
#30580=DIRECTION('ref_axis',(0.707106781186554,0.,0.707106781186541));
#30581=DIRECTION('',(0.707106781186554,0.,0.707106781186541));
#30582=DIRECTION('',(0.,-1.,0.));
#30583=DIRECTION('center_axis',(0.,0.,1.));
#30584=DIRECTION('ref_axis',(-1.,0.,0.));
#30585=DIRECTION('center_axis',(0.,0.,-1.));
#30586=DIRECTION('ref_axis',(1.,0.,0.));
#30587=DIRECTION('',(0.,0.,-1.));
#30588=DIRECTION('center_axis',(0.707106781186541,0.,0.707106781186554));
#30589=DIRECTION('ref_axis',(0.707106781186554,0.,-0.707106781186541));
#30590=DIRECTION('',(-0.707106781186554,0.,0.707106781186541));
#30591=DIRECTION('',(0.707106781186554,0.,-0.707106781186541));
#30592=DIRECTION('center_axis',(0.,0.,1.));
#30593=DIRECTION('ref_axis',(1.,0.,0.));
#30594=DIRECTION('',(0.707106781186554,0.,0.707106781186541));
#30595=DIRECTION('center_axis',(0.,0.,-1.));
#30596=DIRECTION('ref_axis',(1.,0.,0.));
#30597=DIRECTION('center_axis',(-0.707106781186541,0.,0.707106781186554));
#30598=DIRECTION('ref_axis',(0.707106781186554,0.,0.707106781186541));
#30599=DIRECTION('',(0.707106781186554,0.,0.707106781186541));
#30600=DIRECTION('',(0.,-1.,0.));
#30601=DIRECTION('center_axis',(0.,0.,1.));
#30602=DIRECTION('ref_axis',(-1.,0.,0.));
#30603=DIRECTION('center_axis',(0.,0.,-1.));
#30604=DIRECTION('ref_axis',(1.,0.,0.));
#30605=DIRECTION('',(0.,0.,-1.));
#30606=DIRECTION('center_axis',(0.707106781186566,0.,0.707106781186529));
#30607=DIRECTION('ref_axis',(0.707106781186529,0.,-0.707106781186566));
#30608=DIRECTION('',(-0.707106781186529,0.,0.707106781186566));
#30609=DIRECTION('',(0.707106781186529,0.,-0.707106781186566));
#30610=DIRECTION('center_axis',(0.,0.,1.));
#30611=DIRECTION('ref_axis',(1.,-3.22973970800045E-15,0.));
#30612=DIRECTION('',(0.707106781186554,0.,0.707106781186541));
#30613=DIRECTION('center_axis',(0.,0.,-1.));
#30614=DIRECTION('ref_axis',(1.,-3.22973970800045E-15,0.));
#30615=DIRECTION('center_axis',(-0.707106781186566,0.,0.707106781186529));
#30616=DIRECTION('ref_axis',(0.707106781186529,0.,0.707106781186566));
#30617=DIRECTION('',(0.707106781186529,0.,0.707106781186566));
#30618=DIRECTION('',(0.,-1.,0.));
#30619=DIRECTION('center_axis',(0.,0.,1.));
#30620=DIRECTION('ref_axis',(-1.,3.22973970800045E-15,0.));
#30621=DIRECTION('center_axis',(0.,0.,-1.));
#30622=DIRECTION('ref_axis',(1.,-3.22973970800045E-15,0.));
#30623=DIRECTION('',(0.,0.,-1.));
#30624=DIRECTION('',(-0.468387297256998,-0.511424326801133,0.720457144960262));
#30625=DIRECTION('center_axis',(0.,0.,-1.));
#30626=DIRECTION('ref_axis',(1.,1.77635683940025E-15,0.));
#30627=DIRECTION('',(0.,-0.707106781186566,0.707106781186529));
#30628=DIRECTION('',(0.494974746830587,0.504975246918101,-0.707106781186547));
#30629=DIRECTION('center_axis',(0.,0.,1.));
#30630=DIRECTION('ref_axis',(1.,1.77635683940025E-15,0.));
#30631=DIRECTION('center_axis',(0.,0.707106781186541,0.707106781186554));
#30632=DIRECTION('ref_axis',(1.,0.,0.));
#30633=DIRECTION('',(0.,-0.707106781186554,0.707106781186541));
#30634=DIRECTION('',(-1.,0.,0.));
#30635=DIRECTION('center_axis',(0.,0.,-1.));
#30636=DIRECTION('ref_axis',(0.,1.,0.));
#30637=DIRECTION('',(0.707106781186554,0.,0.707106781186541));
#30638=DIRECTION('center_axis',(0.,0.,1.));
#30639=DIRECTION('ref_axis',(0.,1.,0.));
#30640=DIRECTION('center_axis',(-0.707106781186541,0.,0.707106781186554));
#30641=DIRECTION('ref_axis',(0.707106781186554,0.,0.707106781186541));
#30642=DIRECTION('',(0.707106781186554,0.,0.707106781186541));
#30643=DIRECTION('',(0.,-1.,0.));
#30644=DIRECTION('center_axis',(0.,0.,-1.));
#30645=DIRECTION('ref_axis',(-1.,0.,0.));
#30646=DIRECTION('',(0.,0.707106781186554,0.707106781186541));
#30647=DIRECTION('center_axis',(0.,0.,1.));
#30648=DIRECTION('ref_axis',(-1.,0.,0.));
#30649=DIRECTION('center_axis',(0.,-0.707106781186541,0.707106781186554));
#30650=DIRECTION('ref_axis',(1.,0.,0.));
#30651=DIRECTION('',(0.,0.707106781186554,0.707106781186541));
#30652=DIRECTION('center_axis',(0.,0.,-1.));
#30653=DIRECTION('ref_axis',(0.,-1.,0.));
#30654=DIRECTION('',(-0.494974746830587,0.504975246918101,0.707106781186547));
#30655=DIRECTION('',(0.468387297257005,-0.511424326801092,-0.720457144960286));
#30656=DIRECTION('center_axis',(0.,1.,0.));
#30657=DIRECTION('ref_axis',(0.707106781186552,0.,0.707106781186543));
#30658=DIRECTION('center_axis',(0.,-0.792531591590824,-0.609830858788332));
#30659=DIRECTION('ref_axis',(7.33239017272468E-17,-0.609830858788332,0.792531591590824));
#30660=DIRECTION('center_axis',(0.,0.,1.));
#30661=DIRECTION('ref_axis',(-1.,0.,0.));
#30662=DIRECTION('',(0.,0.,1.));
#30663=DIRECTION('center_axis',(-1.,0.,0.));
#30664=DIRECTION('ref_axis',(0.,-1.,0.));
#30665=DIRECTION('',(0.,0.,1.));
#30666=DIRECTION('center_axis',(0.,0.,1.));
#30667=DIRECTION('ref_axis',(0.,1.,0.));
#30668=DIRECTION('',(0.,0.,1.));
#30669=DIRECTION('center_axis',(0.,1.,0.));
#30670=DIRECTION('ref_axis',(-1.,0.,0.));
#30671=DIRECTION('',(0.,0.,1.));
#30672=DIRECTION('center_axis',(-0.707106781186541,0.707106781186554,0.));
#30673=DIRECTION('ref_axis',(0.,0.,1.));
#30674=DIRECTION('',(0.,0.,-1.));
#30675=DIRECTION('',(0.,0.,1.));
#30676=DIRECTION('center_axis',(0.,-1.,0.));
#30677=DIRECTION('ref_axis',(-0.999937018558663,0.,0.0112231419848006));
#30678=DIRECTION('center_axis',(0.,1.,0.));
#30679=DIRECTION('ref_axis',(-0.999937018558664,0.,0.0112231419848006));
#30680=DIRECTION('',(0.659148681788774,0.707106781186549,-0.255974637993922));
#30681=DIRECTION('center_axis',(0.,-1.,0.));
#30682=DIRECTION('ref_axis',(-0.999937018558664,0.,0.0112231419848006));
#30683=DIRECTION('',(-0.658168284632395,-0.706843019174437,0.259205430784961));
#30684=DIRECTION('',(0.658168284632367,-0.70684301917446,-0.259205430784969));
#30685=DIRECTION('center_axis',(0.,1.,0.));
#30686=DIRECTION('ref_axis',(0.,0.,1.));
#30687=DIRECTION('',(1.,0.,0.));
#30688=DIRECTION('',(0.,0.,1.));
#30689=DIRECTION('center_axis',(1.,0.,0.));
#30690=DIRECTION('ref_axis',(0.,1.,0.));
#30691=DIRECTION('',(1.,0.,0.));
#30692=DIRECTION('center_axis',(-1.,0.,0.));
#30693=DIRECTION('ref_axis',(0.,6.12323399573677E-17,1.));
#30694=DIRECTION('center_axis',(0.,-1.,0.));
#30695=DIRECTION('ref_axis',(0.,0.,-1.));
#30696=DIRECTION('',(0.,0.,-1.));
#30697=DIRECTION('center_axis',(-0.70710678118654,-0.683503869536805,0.181169700359153));
#30698=DIRECTION('ref_axis',(0.24819572925489,0.,0.968709904966205));
#30699=DIRECTION('',(0.,-0.256212647338981,-0.966620442233429));
#30700=DIRECTION('',(0.,0.256212647338981,0.966620442233429));
#30701=DIRECTION('center_axis',(-0.70710678118654,-0.683503869536805,0.181169700359153));
#30702=DIRECTION('ref_axis',(-0.662116968503032,0.729946888703702,0.169642741348226));
#30703=DIRECTION('center_axis',(1.,0.,0.));
#30704=DIRECTION('ref_axis',(0.,0.,-1.));
#30705=DIRECTION('',(0.,1.,0.));
#30706=DIRECTION('center_axis',(0.,1.,0.));
#30707=DIRECTION('ref_axis',(-0.999937018558664,0.,0.0112231419848006));
#30708=DIRECTION('center_axis',(-0.707106781186546,0.683503869536799,0.181169700359152));
#30709=DIRECTION('ref_axis',(-0.662116968503027,-0.729946888703707,0.169642741348222));
#30710=DIRECTION('center_axis',(-0.707106781186546,0.683503869536799,0.181169700359152));
#30711=DIRECTION('ref_axis',(0.248195729254886,0.,0.968709904966206));
#30712=DIRECTION('',(0.,0.256212647338981,-0.966620442233429));
#30713=DIRECTION('center_axis',(0.,0.966620442233429,0.256212647338981));
#30714=DIRECTION('ref_axis',(0.,-0.256212647338981,0.966620442233429));
#30715=DIRECTION('',(0.,-0.256212647338981,0.966620442233429));
#30716=DIRECTION('center_axis',(0.,-0.256212647338981,0.966620442233429));
#30717=DIRECTION('ref_axis',(0.707106781186545,0.683503869536801,0.181169700359147));
#30718=DIRECTION('center_axis',(0.,0.256212647338975,-0.966620442233431));
#30719=DIRECTION('ref_axis',(0.,0.966620442233431,0.256212647338975));
#30720=DIRECTION('center_axis',(0.,0.792531591590825,-0.609830858788332));
#30721=DIRECTION('ref_axis',(1.46647803454493E-16,0.609830858788331,0.792531591590825));
#30722=DIRECTION('center_axis',(-1.22056273718388E-14,0.256212647338986,
0.966620442233428));
#30723=DIRECTION('ref_axis',(0.,-0.966620442233428,0.256212647338986));
#30724=DIRECTION('center_axis',(0.,-0.256212647338981,-0.966620442233429));
#30725=DIRECTION('ref_axis',(0.707106781186543,-0.683503869536803,0.181169700359147));
#30726=DIRECTION('',(0.,-0.256212647338981,-0.966620442233429));
#30727=DIRECTION('center_axis',(0.,-0.966620442233429,0.256212647338981));
#30728=DIRECTION('ref_axis',(0.,-0.256212647338981,-0.966620442233429));
#30729=DIRECTION('center_axis',(0.,0.,1.));
#30730=DIRECTION('ref_axis',(0.707106781186545,0.70710678118655,0.));
#30731=DIRECTION('center_axis',(0.,0.,-1.));
#30732=DIRECTION('ref_axis',(0.,1.,0.));
#30733=DIRECTION('center_axis',(0.,-0.707106781186549,0.707106781186546));
#30734=DIRECTION('ref_axis',(0.,-0.707106781186546,-0.707106781186549));
#30735=DIRECTION('center_axis',(0.,1.,0.));
#30736=DIRECTION('ref_axis',(0.707106781186552,0.,0.707106781186543));
#30737=DIRECTION('center_axis',(-2.09345661157836E-15,-0.707106781186549,
-0.707106781186546));
#30738=DIRECTION('ref_axis',(2.09345661157836E-15,-0.707106781186546,0.707106781186549));
#30739=DIRECTION('center_axis',(-1.,0.,0.));
#30740=DIRECTION('ref_axis',(0.,0.,1.));
#30741=DIRECTION('center_axis',(0.,0.,1.));
#30742=DIRECTION('ref_axis',(0.,-1.,0.));
#30743=DIRECTION('center_axis',(0.,0.,-1.));
#30744=DIRECTION('ref_axis',(0.707106781186545,-0.70710678118655,0.));
#30745=DIRECTION('center_axis',(0.,1.,0.));
#30746=DIRECTION('ref_axis',(0.707106781186552,0.,0.707106781186543));
#30747=DIRECTION('center_axis',(0.,0.,1.));
#30748=DIRECTION('ref_axis',(1.,1.77635683940025E-15,0.));
#30749=DIRECTION('center_axis',(1.,0.,0.));
#30750=DIRECTION('ref_axis',(0.,0.,-1.));
#30751=DIRECTION('center_axis',(1.,0.,0.));
#30752=DIRECTION('ref_axis',(0.,-1.,0.));
#30753=DIRECTION('center_axis',(1.,0.,0.));
#30754=DIRECTION('ref_axis',(0.,-1.,0.));
#30755=DIRECTION('center_axis',(1.,0.,0.));
#30756=DIRECTION('ref_axis',(0.,-1.,0.));
#30757=DIRECTION('center_axis',(1.,0.,0.));
#30758=DIRECTION('ref_axis',(0.,-1.,0.));
#30759=DIRECTION('center_axis',(-1.,0.,0.));
#30760=DIRECTION('ref_axis',(0.,0.,1.));
#30761=DIRECTION('',(-0.515038074910054,-1.04972719113862E-16,-0.857167300702112));
#30762=DIRECTION('center_axis',(-1.,0.,0.));
#30763=DIRECTION('ref_axis',(0.,0.,1.));
#30764=DIRECTION('',(-0.515038074910054,-1.04972719113862E-16,-0.857167300702112));
#30765=DIRECTION('center_axis',(-1.,0.,0.));
#30766=DIRECTION('ref_axis',(0.,0.,1.));
#30767=DIRECTION('',(-0.515038074910054,-1.04972719113862E-16,-0.857167300702112));
#30768=DIRECTION('center_axis',(-1.,0.,0.));
#30769=DIRECTION('ref_axis',(0.,0.,1.));
#30770=DIRECTION('',(-0.515038074910054,-1.04972719113862E-16,-0.857167300702112));
#30771=DIRECTION('center_axis',(0.,0.,1.));
#30772=DIRECTION('ref_axis',(1.,0.,0.));
#30773=DIRECTION('center_axis',(0.,0.,1.));
#30774=DIRECTION('ref_axis',(1.,0.,0.));
#30775=DIRECTION('center_axis',(0.,0.,1.));
#30776=DIRECTION('ref_axis',(1.,0.,0.));
#30777=DIRECTION('',(0.,0.,1.));
#30778=DIRECTION('center_axis',(0.,0.,1.));
#30779=DIRECTION('ref_axis',(1.,0.,0.));
#30780=DIRECTION('',(0.,0.,1.));
#30781=DIRECTION('center_axis',(0.,0.,1.));
#30782=DIRECTION('ref_axis',(1.,0.,0.));
#30783=DIRECTION('center_axis',(0.,0.,1.));
#30784=DIRECTION('ref_axis',(1.,0.,0.));
#30785=DIRECTION('center_axis',(0.,0.,1.));
#30786=DIRECTION('ref_axis',(1.,0.,0.));
#30787=DIRECTION('center_axis',(0.,0.,1.));
#30788=DIRECTION('ref_axis',(1.,0.,0.));
#30789=DIRECTION('',(0.,0.,1.));
#30790=DIRECTION('center_axis',(1.,0.,0.));
#30791=DIRECTION('ref_axis',(0.,1.,0.));
#30792=DIRECTION('center_axis',(1.,0.,0.));
#30793=DIRECTION('ref_axis',(0.,1.,0.));
#30794=DIRECTION('',(1.,0.,0.));
#30795=DIRECTION('center_axis',(-1.,0.,0.));
#30796=DIRECTION('ref_axis',(0.,0.,1.));
#37039=CARTESIAN_POINT('',(0.,0.,0.));
#37040=CARTESIAN_POINT('Origin',(33.5,-5.31299340340571E-17,33.4823223304703));
#37041=CARTESIAN_POINT('',(35.15,-2.02066721859314E-16,33.5));
#37042=CARTESIAN_POINT('Origin',(33.5,0.,33.5));
#37043=CARTESIAN_POINT('',(35.2353553390593,2.12519736136229E-16,33.4646446609407));
#37044=CARTESIAN_POINT('',(35.1926776695297,2.07293228997771E-16,33.4823223304703));
#37045=CARTESIAN_POINT('',(31.7646446609407,-2.12519736136228E-16,33.4646446609407));
#37046=CARTESIAN_POINT('Origin',(33.5,-1.06259868068114E-16,33.4646446609407));
#37047=CARTESIAN_POINT('Origin',(33.5,-1.06259868068114E-16,33.4646446609407));
#37048=CARTESIAN_POINT('Origin',(33.5,0.,33.45));
#37049=CARTESIAN_POINT('',(31.7353553390593,-2.16106643565346E-16,33.4353553390593));
#37050=CARTESIAN_POINT('',(31.75,-2.14313189850787E-16,33.45));
#37051=CARTESIAN_POINT('',(35.2646446609407,-2.16106643565346E-16,33.4353553390593));
#37052=CARTESIAN_POINT('Origin',(33.5,-1.08053321782673E-16,33.4353553390593));
#37053=CARTESIAN_POINT('Origin',(33.5,-1.08053321782673E-16,33.4353553390593));
#37054=CARTESIAN_POINT('Origin',(33.5,0.,33.5));
#37055=CARTESIAN_POINT('',(32.895,-7.40911313484154E-17,33.5));
#37056=CARTESIAN_POINT('Origin',(33.5,0.,33.5));
#37057=CARTESIAN_POINT('Origin',(33.5,-5.40266608913365E-17,33.3926776695297));
#37058=CARTESIAN_POINT('',(35.3,2.20436423846523E-16,33.35));
#37059=CARTESIAN_POINT('',(35.2823223304703,2.18271533705935E-16,33.3926776695297));
#37060=CARTESIAN_POINT('',(31.7,-2.20436423846523E-16,33.35));
#37061=CARTESIAN_POINT('Origin',(33.5,0.,33.35));
#37062=CARTESIAN_POINT('Origin',(33.5,0.,33.35));
#37063=CARTESIAN_POINT('Origin',(33.5,0.,29.95));
#37064=CARTESIAN_POINT('',(31.7,-2.9062945342485E-16,32.));
#37065=CARTESIAN_POINT('',(31.7,-2.20436423846523E-16,29.95));
#37066=CARTESIAN_POINT('',(33.5,-1.8,31.6971145840745));
#37067=CARTESIAN_POINT('Ctrl Pts',(33.5,-1.8,31.6971145840745));
#37068=CARTESIAN_POINT('Ctrl Pts',(33.3860566581303,-1.8,31.6971145840745));
#37069=CARTESIAN_POINT('Ctrl Pts',(33.2685178334622,-1.78900665408164,31.700965713284));
#37070=CARTESIAN_POINT('Ctrl Pts',(33.0352764413812,-1.74303207564077,31.716553300941));
#37071=CARTESIAN_POINT('Ctrl Pts',(32.9195702475634,-1.70806396550477,31.7282741932561));
#37072=CARTESIAN_POINT('Ctrl Pts',(32.6981116334826,-1.61596921995123,31.7574686694119));
#37073=CARTESIAN_POINT('Ctrl Pts',(32.5921667861828,-1.55876952413463,31.7749340986735));
#37074=CARTESIAN_POINT('Ctrl Pts',(32.3964416611508,-1.42691365092969,31.8121191258143));
#37075=CARTESIAN_POINT('Ctrl Pts',(32.3066617865707,-1.3522461988423,31.8318008558006));
#37076=CARTESIAN_POINT('Ctrl Pts',(32.1477879055675,-1.19337231783909,31.8695928089871));
#37077=CARTESIAN_POINT('Ctrl Pts',(32.0731245394823,-1.10360856854857,31.8890590514301));
#37078=CARTESIAN_POINT('Ctrl Pts',(31.9412537861583,-0.907874271943785,
31.9254652923589));
#37079=CARTESIAN_POINT('Ctrl Pts',(31.8840366362977,-0.801904114450162,
31.9423720162283));
#37080=CARTESIAN_POINT('Ctrl Pts',(31.7919223266258,-0.580395123714868,
31.9704300444786));
#37081=CARTESIAN_POINT('Ctrl Pts',(31.7569520118305,-0.464664625832372,
31.9815821366528));
#37082=CARTESIAN_POINT('Ctrl Pts',(31.7109845655851,-0.231415814089425,
31.9963717720298));
#37083=CARTESIAN_POINT('Ctrl Pts',(31.7,-0.113894433434802,32.));
#37084=CARTESIAN_POINT('Ctrl Pts',(31.7,-1.66533453693773E-16,32.));
#37085=CARTESIAN_POINT('Ctrl Pts',(31.7,-2.22044604925031E-16,32.));
#37086=CARTESIAN_POINT('Ctrl Pts',(31.7,0.113894433434802,32.));
#37087=CARTESIAN_POINT('Ctrl Pts',(31.7109845655851,0.231415814089425,31.9963717720298));
#37088=CARTESIAN_POINT('Ctrl Pts',(31.7569520118305,0.464664625832373,31.9815821366528));
#37089=CARTESIAN_POINT('Ctrl Pts',(31.7919223266258,0.58039512371487,31.9704300444786));
#37090=CARTESIAN_POINT('Ctrl Pts',(31.8840366362977,0.801904114450163,31.9423720162283));
#37091=CARTESIAN_POINT('Ctrl Pts',(31.9412537861583,0.907874271943785,31.9254652923589));
#37092=CARTESIAN_POINT('Ctrl Pts',(32.0731245394823,1.10360856854856,31.8890590514301));
#37093=CARTESIAN_POINT('Ctrl Pts',(32.1477879055675,1.19337231783909,31.8695928089871));
#37094=CARTESIAN_POINT('Ctrl Pts',(32.3066617865707,1.3522461988423,31.8318008558006));
#37095=CARTESIAN_POINT('Ctrl Pts',(32.3964416611508,1.4269136509297,31.8121191258143));
#37096=CARTESIAN_POINT('Ctrl Pts',(32.5921667861828,1.55876952413463,31.7749340986735));
#37097=CARTESIAN_POINT('Ctrl Pts',(32.6981116334826,1.61596921995123,31.7574686694119));
#37098=CARTESIAN_POINT('Ctrl Pts',(32.9195702475634,1.70806396550477,31.7282741932561));
#37099=CARTESIAN_POINT('Ctrl Pts',(33.0352764413812,1.74303207564077,31.716553300941));
#37100=CARTESIAN_POINT('Ctrl Pts',(33.2685178334622,1.78900665408164,31.700965713284));
#37101=CARTESIAN_POINT('Ctrl Pts',(33.3860566581303,1.8,31.6971145840745));
#37102=CARTESIAN_POINT('Ctrl Pts',(33.6139433418697,1.8,31.6971145840745));
#37103=CARTESIAN_POINT('Ctrl Pts',(33.7314821665378,1.78900665408164,31.700965713284));
#37104=CARTESIAN_POINT('Ctrl Pts',(33.9647235586188,1.74303207564077,31.716553300941));
#37105=CARTESIAN_POINT('Ctrl Pts',(34.0804297524366,1.70806396550477,31.7282741932561));
#37106=CARTESIAN_POINT('Ctrl Pts',(34.3018883665174,1.61596921995123,31.7574686694119));
#37107=CARTESIAN_POINT('Ctrl Pts',(34.4078332138172,1.55876952413463,31.7749340986735));
#37108=CARTESIAN_POINT('Ctrl Pts',(34.6035583388492,1.4269136509297,31.8121191258143));
#37109=CARTESIAN_POINT('Ctrl Pts',(34.6933382134293,1.3522461988423,31.8318008558006));
#37110=CARTESIAN_POINT('Ctrl Pts',(34.8522120944325,1.19337231783909,31.8695928089871));
#37111=CARTESIAN_POINT('Ctrl Pts',(34.9268754605177,1.10360856854856,31.8890590514301));
#37112=CARTESIAN_POINT('Ctrl Pts',(35.0587462138417,0.907874271943785,31.9254652923589));
#37113=CARTESIAN_POINT('Ctrl Pts',(35.1159633637023,0.801904114450164,31.9423720162283));
#37114=CARTESIAN_POINT('Ctrl Pts',(35.2080776733742,0.58039512371487,31.9704300444786));
#37115=CARTESIAN_POINT('Ctrl Pts',(35.2430479881695,0.464664625832375,31.9815821366528));
#37116=CARTESIAN_POINT('Ctrl Pts',(35.2890154344149,0.231415814089427,31.9963717720298));
#37117=CARTESIAN_POINT('Ctrl Pts',(35.3,0.113894433434802,32.));
#37118=CARTESIAN_POINT('Ctrl Pts',(35.3,-0.113894433434802,32.));
#37119=CARTESIAN_POINT('Ctrl Pts',(35.2890154344149,-0.231415814089426,
31.9963717720298));
#37120=CARTESIAN_POINT('Ctrl Pts',(35.2430479881695,-0.464664625832374,
31.9815821366528));
#37121=CARTESIAN_POINT('Ctrl Pts',(35.2080776733742,-0.58039512371487,31.9704300444786));
#37122=CARTESIAN_POINT('Ctrl Pts',(35.1159633637023,-0.801904114450163,
31.9423720162283));
#37123=CARTESIAN_POINT('Ctrl Pts',(35.0587462138417,-0.907874271943786,
31.9254652923589));
#37124=CARTESIAN_POINT('Ctrl Pts',(34.9268754605177,-1.10360856854856,31.8890590514301));
#37125=CARTESIAN_POINT('Ctrl Pts',(34.8522120944325,-1.19337231783909,31.8695928089871));
#37126=CARTESIAN_POINT('Ctrl Pts',(34.6933382134293,-1.3522461988423,31.8318008558006));
#37127=CARTESIAN_POINT('Ctrl Pts',(34.6035583388492,-1.4269136509297,31.8121191258143));
#37128=CARTESIAN_POINT('Ctrl Pts',(34.4078332138172,-1.55876952413463,31.7749340986735));
#37129=CARTESIAN_POINT('Ctrl Pts',(34.3018883665174,-1.61596921995123,31.7574686694119));
#37130=CARTESIAN_POINT('Ctrl Pts',(34.0804297524366,-1.70806396550477,31.7282741932561));
#37131=CARTESIAN_POINT('Ctrl Pts',(33.9647235586188,-1.74303207564076,31.716553300941));
#37132=CARTESIAN_POINT('Ctrl Pts',(33.7314821665378,-1.78900665408164,31.700965713284));
#37133=CARTESIAN_POINT('Ctrl Pts',(33.6139433418697,-1.8,31.6971145840745));
#37134=CARTESIAN_POINT('Ctrl Pts',(33.5,-1.8,31.6971145840745));
#37135=CARTESIAN_POINT('Origin',(8.025,3.53553390593274,30.0355339059327));
#37136=CARTESIAN_POINT('',(8.,3.60696374383365,30.3832734323853));
#37137=CARTESIAN_POINT('',(8.,3.8832734323853,30.1069637438337));
#37138=CARTESIAN_POINT('Ctrl Pts',(8.,3.60696374383365,30.3832734323853));
#37139=CARTESIAN_POINT('Ctrl Pts',(8.01789140164846,3.66596515189423,30.3528888836206));
#37140=CARTESIAN_POINT('Ctrl Pts',(8.0275,3.72132986391805,30.3128928896246));
#37141=CARTESIAN_POINT('Ctrl Pts',(8.0275,3.81289288962462,30.2213298639181));
#37142=CARTESIAN_POINT('Ctrl Pts',(8.01789140164846,3.85288888362064,30.1659651518942));
#37143=CARTESIAN_POINT('Ctrl Pts',(8.,3.8832734323853,30.1069637438336));
#37144=CARTESIAN_POINT('',(8.,3.53553390593274,30.3905339059327));
#37145=CARTESIAN_POINT('Origin',(8.,3.53553390593274,30.0355339059327));
#37146=CARTESIAN_POINT('',(8.05,3.53553390593274,30.3405339059327));
#37147=CARTESIAN_POINT('',(8.025,3.53553390593274,30.3655339059327));
#37148=CARTESIAN_POINT('',(8.05,3.53553390593274,29.7305339059327));
#37149=CARTESIAN_POINT('Origin',(8.05,3.53553390593274,30.0355339059327));
#37150=CARTESIAN_POINT('Origin',(8.05,3.53553390593274,30.0355339059327));
#37151=CARTESIAN_POINT('Origin',(8.,3.53553390593274,30.0355339059327));
#37152=CARTESIAN_POINT('Origin',(8.1,0.,26.5));
#37153=CARTESIAN_POINT('',(8.2,5.5,26.5));
#37154=CARTESIAN_POINT('',(8.2,-5.5,26.5));
#37155=CARTESIAN_POINT('Origin',(8.2,0.,26.5));
#37156=CARTESIAN_POINT('Origin',(8.2,0.,26.5));
#37157=CARTESIAN_POINT('',(8.,5.3,26.5));
#37158=CARTESIAN_POINT('',(8.1,5.4,26.5));
#37159=CARTESIAN_POINT('Origin',(8.,0.,26.5));
#37160=CARTESIAN_POINT('',(8.,-3.60696374383365,30.3832734323853));
#37161=CARTESIAN_POINT('Origin',(8.,0.,26.5));
#37162=CARTESIAN_POINT('',(8.,-3.8832734323853,30.1069637438337));
#37163=CARTESIAN_POINT('Ctrl Pts',(8.,-3.8832734323853,30.1069637438337));
#37164=CARTESIAN_POINT('Ctrl Pts',(8.01789140164973,-3.85288888361848,30.1659651518984));
#37165=CARTESIAN_POINT('Ctrl Pts',(8.0275,-3.81289288959515,30.2213298639475));
#37166=CARTESIAN_POINT('Ctrl Pts',(8.0275,-3.72132986394751,30.3128928895952));
#37167=CARTESIAN_POINT('Ctrl Pts',(8.01789140164973,-3.66596515189844,30.3528888836185));
#37168=CARTESIAN_POINT('Ctrl Pts',(8.,-3.60696374383365,30.3832734323853));
#37169=CARTESIAN_POINT('',(8.,-3.8832734323853,22.8930362561663));
#37170=CARTESIAN_POINT('Origin',(8.,0.,26.5));
#37171=CARTESIAN_POINT('',(8.,-3.60696374383365,22.6167265676147));
#37172=CARTESIAN_POINT('Ctrl Pts',(8.,-3.60696374383365,22.6167265676147));
#37173=CARTESIAN_POINT('Ctrl Pts',(8.01789141230059,-3.66596518702231,22.6471111344696));
#37174=CARTESIAN_POINT('Ctrl Pts',(8.0275,-3.72133011029548,22.6871073567528));
#37175=CARTESIAN_POINT('Ctrl Pts',(8.0275,-3.81289264324719,22.7786698897045));
#37176=CARTESIAN_POINT('Ctrl Pts',(8.01789141230058,-3.85288886553039,22.8340348129777));
#37177=CARTESIAN_POINT('Ctrl Pts',(8.,-3.8832734323853,22.8930362561663));
#37178=CARTESIAN_POINT('',(8.,3.60696374383366,22.6167265676147));
#37179=CARTESIAN_POINT('Origin',(8.,0.,26.5));
#37180=CARTESIAN_POINT('',(8.,3.88327343238529,22.8930362561663));
#37181=CARTESIAN_POINT('Ctrl Pts',(8.,3.88327343238529,22.8930362561663));
#37182=CARTESIAN_POINT('Ctrl Pts',(8.01789140164846,3.85288888362063,22.8340348481058));
#37183=CARTESIAN_POINT('Ctrl Pts',(8.0275,3.81289288962461,22.7786701360819));
#37184=CARTESIAN_POINT('Ctrl Pts',(8.0275,3.72132986391806,22.6871071103754));
#37185=CARTESIAN_POINT('Ctrl Pts',(8.01789140164846,3.66596515189424,22.6471111163794));
#37186=CARTESIAN_POINT('Ctrl Pts',(8.,3.60696374383366,22.6167265676147));
#37187=CARTESIAN_POINT('Origin',(8.,0.,26.5));
#37188=CARTESIAN_POINT('Origin',(8.685,3.53553390593274,30.0355339059327));
#37189=CARTESIAN_POINT('',(9.4,3.53553390593274,29.7305339059327));
#37190=CARTESIAN_POINT('Origin',(9.4,3.53553390593274,30.0355339059327));
#37191=CARTESIAN_POINT('',(8.685,3.53553390593274,29.7305339059327));
#37192=CARTESIAN_POINT('Origin',(8.025,3.53553390593274,22.9644660940673));
#37193=CARTESIAN_POINT('',(8.,3.53553390593274,22.6094660940673));
#37194=CARTESIAN_POINT('Origin',(8.,3.53553390593274,22.9644660940673));
#37195=CARTESIAN_POINT('',(8.05,3.53553390593274,22.6594660940673));
#37196=CARTESIAN_POINT('',(8.025,3.53553390593274,22.6344660940673));
#37197=CARTESIAN_POINT('Origin',(8.05,3.53553390593274,22.9644660940673));
#37198=CARTESIAN_POINT('Origin',(8.,3.53553390593274,22.9644660940673));
#37199=CARTESIAN_POINT('Origin',(8.685,3.53553390593274,22.9644660940673));
#37200=CARTESIAN_POINT('',(9.4,3.53553390593274,22.6594660940673));
#37201=CARTESIAN_POINT('Origin',(9.4,3.53553390593274,22.9644660940673));
#37202=CARTESIAN_POINT('',(8.685,3.53553390593274,22.6594660940673));
#37203=CARTESIAN_POINT('Origin',(21.025,-5.55,4.225));
#37204=CARTESIAN_POINT('',(21.025,10.975,4.225));
#37205=CARTESIAN_POINT('',(21.05,10.95,4.2));
#37206=CARTESIAN_POINT('',(24.4416666666667,7.55833333333329,0.808333333333354));
#37207=CARTESIAN_POINT('',(21.05,-10.95,4.2));
#37208=CARTESIAN_POINT('',(21.05,-5.55,4.2));
#37209=CARTESIAN_POINT('',(21.025,-10.975,4.225));
#37210=CARTESIAN_POINT('',(20.925,-11.075,4.325));
#37211=CARTESIAN_POINT('',(21.,-10.95,4.25));
#37212=CARTESIAN_POINT('',(20.125,-10.075,5.12499999999999));
#37213=CARTESIAN_POINT('',(21.,10.95,4.25));
#37214=CARTESIAN_POINT('',(21.,-5.55,4.25));
#37215=CARTESIAN_POINT('',(18.275,8.22499999999997,6.97499999999998));
#37216=CARTESIAN_POINT('Origin',(20.,0.,4.2));
#37217=CARTESIAN_POINT('',(30.,10.95,4.2));
#37218=CARTESIAN_POINT('',(25.,10.95,4.2));
#37219=CARTESIAN_POINT('',(30.665,10.6784357007116,4.2));
#37220=CARTESIAN_POINT('Origin',(30.,10.,4.2));
#37221=CARTESIAN_POINT('',(30.7,10.6423370590817,4.2));
#37222=CARTESIAN_POINT('Ctrl Pts',(30.7,10.6423370590817,4.2));
#37223=CARTESIAN_POINT('Ctrl Pts',(30.6885903428187,10.6546728503156,4.2));
#37224=CARTESIAN_POINT('Ctrl Pts',(30.6769830660874,10.6666899465601,4.2));
#37225=CARTESIAN_POINT('Ctrl Pts',(30.665,10.6784357007116,4.2));
#37226=CARTESIAN_POINT('',(30.7,-10.6423370590817,4.2));
#37227=CARTESIAN_POINT('',(30.7,0.,4.2));
#37228=CARTESIAN_POINT('',(30.665,-10.6784357007116,4.2));
#37229=CARTESIAN_POINT('Ctrl Pts',(30.665,-10.6784357007116,4.2));
#37230=CARTESIAN_POINT('Ctrl Pts',(30.6769830660874,-10.6666899465601,4.2));
#37231=CARTESIAN_POINT('Ctrl Pts',(30.6885903428187,-10.6546728503156,4.2));
#37232=CARTESIAN_POINT('Ctrl Pts',(30.7,-10.6423370590817,4.2));
#37233=CARTESIAN_POINT('',(30.,-10.95,4.2));
#37234=CARTESIAN_POINT('Origin',(30.,-10.,4.2));
#37235=CARTESIAN_POINT('',(15.,-10.95,4.2));
#37236=CARTESIAN_POINT('',(28.4,9.,4.2));
#37237=CARTESIAN_POINT('',(28.4,9.4,4.2));
#37238=CARTESIAN_POINT('',(28.4,4.5,4.2));
#37239=CARTESIAN_POINT('',(29.6,9.,4.2));
#37240=CARTESIAN_POINT('Origin',(29.,9.,4.2));
#37241=CARTESIAN_POINT('',(29.6,9.4,4.2));
#37242=CARTESIAN_POINT('',(29.6,4.7,4.2));
#37243=CARTESIAN_POINT('Origin',(29.,9.4,4.2));
#37244=CARTESIAN_POINT('',(28.4,-9.4,4.2));
#37245=CARTESIAN_POINT('',(28.4,-9.,4.2));
#37246=CARTESIAN_POINT('',(28.4,-4.7,4.2));
#37247=CARTESIAN_POINT('',(29.6,-9.4,4.2));
#37248=CARTESIAN_POINT('Origin',(29.,-9.4,4.2));
#37249=CARTESIAN_POINT('',(29.6,-9.,4.2));
#37250=CARTESIAN_POINT('',(29.6,-4.5,4.2));
#37251=CARTESIAN_POINT('Origin',(29.,-9.,4.2));
#37252=CARTESIAN_POINT('Origin',(25.,10.975,4.225));
#37253=CARTESIAN_POINT('',(21.05,11.,4.25));
#37254=CARTESIAN_POINT('',(21.05,11.,4.25));
#37255=CARTESIAN_POINT('',(30.,11.,4.25));
#37256=CARTESIAN_POINT('',(25.,11.,4.25));
#37257=CARTESIAN_POINT('',(30.,11.,4.25));
#37258=CARTESIAN_POINT('Origin',(21.025,10.975,4.2));
#37259=CARTESIAN_POINT('',(21.,10.95,4.8));
#37260=CARTESIAN_POINT('',(21.,10.95,4.2));
#37261=CARTESIAN_POINT('',(21.05,11.,4.85));
#37262=CARTESIAN_POINT('',(21.,10.95,4.8));
#37263=CARTESIAN_POINT('',(21.05,11.,4.2));
#37264=CARTESIAN_POINT('Origin',(35.9823223304703,0.,26.5));
#37265=CARTESIAN_POINT('',(35.9646446609407,5.33535533905933,26.5));
#37266=CARTESIAN_POINT('Origin',(35.9646446609407,0.,26.5));
#37267=CARTESIAN_POINT('',(36.,5.25,26.5));
#37268=CARTESIAN_POINT('',(35.9823223304703,5.29267766952966,26.5));
#37269=CARTESIAN_POINT('Origin',(36.,0.,26.5));
#37270=CARTESIAN_POINT('Origin',(35.9,0.,26.5));
#37271=CARTESIAN_POINT('',(35.8353553390593,5.46464466094067,26.5));
#37272=CARTESIAN_POINT('',(35.9,5.4,26.5));
#37273=CARTESIAN_POINT('Origin',(35.8353553390593,0.,26.5));
#37274=CARTESIAN_POINT('Origin',(36.,0.,26.5));
#37275=CARTESIAN_POINT('',(36.,-3.5,26.5));
#37276=CARTESIAN_POINT('Origin',(36.,0.,26.5));
#37277=CARTESIAN_POINT('Ctrl Pts',(34.5,-0.749563950038172,21.0513163163198));
#37278=CARTESIAN_POINT('Ctrl Pts',(34.6078091511127,-0.749563950038172,
21.0513163163198));
#37279=CARTESIAN_POINT('Ctrl Pts',(34.7811032097204,-0.711754547708119,
21.0458589692126));
#37280=CARTESIAN_POINT('Ctrl Pts',(34.974965121707,-0.587314921207312,21.0311479468387));
#37281=CARTESIAN_POINT('Ctrl Pts',(35.0549239124764,-0.507046229905794,
21.0232925177222));
#37282=CARTESIAN_POINT('Ctrl Pts',(35.0977756120755,-0.452152037495066,
21.0186704724503));
#37283=CARTESIAN_POINT('Ctrl Pts',(35.1143542325059,-0.429612298109788,
21.0168443285933));
#37284=CARTESIAN_POINT('Ctrl Pts',(35.1340422591755,-0.400351661687876,
21.0146094007192));
#37285=CARTESIAN_POINT('Ctrl Pts',(35.1557767361487,-0.363704460367538,
21.0120527916887));
#37286=CARTESIAN_POINT('Ctrl Pts',(35.1820502322802,-0.313074653150546,
21.0088643148667));
#37287=CARTESIAN_POINT('Ctrl Pts',(35.2039675401431,-0.260041744395718,
21.0060858902635));
#37288=CARTESIAN_POINT('Ctrl Pts',(35.2212309037757,-0.205721880481172,
21.0038401171032));
#37289=CARTESIAN_POINT('Ctrl Pts',(35.2563431722199,-0.0671819342670894,
20.9991778701227));
#37290=CARTESIAN_POINT('Ctrl Pts',(35.2560871656414,0.0626491158681729,
20.9991981622569));
#37291=CARTESIAN_POINT('Ctrl Pts',(35.2245604862986,0.191862595129649,21.0033883099402));
#37292=CARTESIAN_POINT('Ctrl Pts',(35.214068499096,0.228356974265122,21.004762450079));
#37293=CARTESIAN_POINT('Ctrl Pts',(35.1923007590141,0.291280650338835,21.0075819713019));
#37294=CARTESIAN_POINT('Ctrl Pts',(35.0993946204602,0.481448989298802,21.0190440514598));
#37295=CARTESIAN_POINT('Ctrl Pts',(34.9566260210823,0.614115291433095,21.0340667746151));
#37296=CARTESIAN_POINT('Ctrl Pts',(34.8005645030701,0.686149513350896,21.043032043578));
#37297=CARTESIAN_POINT('Ctrl Pts',(34.7653478169603,0.700689089135733,21.0448800812064));
#37298=CARTESIAN_POINT('Ctrl Pts',(34.702486674947,0.722760619862234,21.0477448745898));
#37299=CARTESIAN_POINT('Ctrl Pts',(34.5716817460195,0.751594137177719,21.0516605025898));
#37300=CARTESIAN_POINT('Ctrl Pts',(34.4466588488531,0.751912455450576,21.0516805007024));
#37301=CARTESIAN_POINT('Ctrl Pts',(34.2979168099864,0.724426508507403,21.0479597951114));
#37302=CARTESIAN_POINT('Ctrl Pts',(34.1711411964527,0.680510140463003,21.0421401113897));
#37303=CARTESIAN_POINT('Ctrl Pts',(34.0254400152268,0.587512193866294,21.0312041853341));
#37304=CARTESIAN_POINT('Ctrl Pts',(33.9119242783867,0.473659340333228,21.019990938314));
#37305=CARTESIAN_POINT('Ctrl Pts',(33.8341349430927,0.352541117917839,21.0109182636443));
#37306=CARTESIAN_POINT('Ctrl Pts',(33.7987498653191,0.266554791315046,21.0064207443541));
#37307=CARTESIAN_POINT('Ctrl Pts',(33.785196053886,0.225933611733011,21.0046676361538));
#37308=CARTESIAN_POINT('Ctrl Pts',(33.7790286911615,0.205467311567983,21.0038613997373));
#37309=CARTESIAN_POINT('Ctrl Pts',(33.7743776719825,0.188304504278709,21.0032490851194));
#37310=CARTESIAN_POINT('Ctrl Pts',(33.7713876543967,0.17624582215462,21.00285311147));
#37311=CARTESIAN_POINT('Ctrl Pts',(33.7697534967433,0.169351646984093,21.0026362335653));
#37312=CARTESIAN_POINT('Ctrl Pts',(33.7436322538446,0.0552211959972136,
20.9991614986988));
#37313=CARTESIAN_POINT('Ctrl Pts',(33.743587569203,-0.0671233551084263,
20.9991689935559));
#37314=CARTESIAN_POINT('Ctrl Pts',(33.7787073248947,-0.20567073339148,21.0038317959733));
#37315=CARTESIAN_POINT('Ctrl Pts',(33.7959736390573,-0.259995325676423,
21.0060780038898));
#37316=CARTESIAN_POINT('Ctrl Pts',(33.8233767787127,-0.326253771531467,
21.0095516426503));
#37317=CARTESIAN_POINT('Ctrl Pts',(33.8580412322199,-0.388632549296444,
21.0137091580996));
#37318=CARTESIAN_POINT('Ctrl Pts',(33.8856030358547,-0.42960122555939,21.0168381467451));
#37319=CARTESIAN_POINT('Ctrl Pts',(33.9021823878193,-0.452140301878644,
21.0186643472973));
#37320=CARTESIAN_POINT('Ctrl Pts',(33.945034720446,-0.507035206264715,21.0232865152258));
#37321=CARTESIAN_POINT('Ctrl Pts',(34.02500542513,-0.587306740554846,21.0311436542917));
#37322=CARTESIAN_POINT('Ctrl Pts',(34.2188700233853,-0.711747372551822,
21.0458550828561));
#37323=CARTESIAN_POINT('Ctrl Pts',(34.3921908488873,-0.749563950038174,
21.0513163163198));
#37324=CARTESIAN_POINT('Ctrl Pts',(34.5,-0.749563950038174,21.0513163163198));
#37325=CARTESIAN_POINT('Ctrl Pts',(34.5,-0.733042633358783,21.0657866512817));
#37326=CARTESIAN_POINT('Ctrl Pts',(34.6057023393761,-0.733042633358783,
21.0657866512817));
#37327=CARTESIAN_POINT('Ctrl Pts',(34.7755983155706,-0.69581787485872,21.060547064769));
#37328=CARTESIAN_POINT('Ctrl Pts',(34.9652246436437,-0.573673233549097,
21.0464470738094));
#37329=CARTESIAN_POINT('Ctrl Pts',(35.0432940001379,-0.495046067925316,
21.0389275943025));
#37330=CARTESIAN_POINT('Ctrl Pts',(35.0850937946794,-0.441336105285769,
21.0345060806934));
#37331=CARTESIAN_POINT('Ctrl Pts',(35.1012616050954,-0.419288232709881,
21.0327594496866));
#37332=CARTESIAN_POINT('Ctrl Pts',(35.1204550010736,-0.390676354751433,
21.0306223291988));
#37333=CARTESIAN_POINT('Ctrl Pts',(35.1416337966199,-0.354858778393741,
21.028178358288));
#37334=CARTESIAN_POINT('Ctrl Pts',(35.1672245914793,-0.305397290800612,
21.0251312396614));
#37335=CARTESIAN_POINT('Ctrl Pts',(35.1885584093061,-0.253620878979568,
21.0224771785701));
#37336=CARTESIAN_POINT('Ctrl Pts',(35.2053550452028,-0.200615260478044,
21.0203325632711));
#37337=CARTESIAN_POINT('Ctrl Pts',(35.2395058919798,-0.0654667973481286,
21.015881422341));
#37338=CARTESIAN_POINT('Ctrl Pts',(35.2392542870293,0.0610529003734771,
21.015901035455));
#37339=CARTESIAN_POINT('Ctrl Pts',(35.2085910301353,0.187098413030655,21.0199014530354));
#37340=CARTESIAN_POINT('Ctrl Pts',(35.1983841264211,0.222704517693513,21.0212135528815));
#37341=CARTESIAN_POINT('Ctrl Pts',(35.1772017415125,0.284115878094912,21.0239064472591));
#37342=CARTESIAN_POINT('Ctrl Pts',(35.086739809034,0.469851258313408,21.0348573742634));
#37343=CARTESIAN_POINT('Ctrl Pts',(34.9473718771303,0.599947262996566,21.0492416495909));
#37344=CARTESIAN_POINT('Ctrl Pts',(34.7945686206459,0.670705966532925,21.0578389402555));
#37345=CARTESIAN_POINT('Ctrl Pts',(34.7600803705086,0.684991273798064,21.0596112517484));
#37346=CARTESIAN_POINT('Ctrl Pts',(34.6985001107118,0.706684122867952,21.0623592585023));
#37347=CARTESIAN_POINT('Ctrl Pts',(34.5702945224947,0.73504254109294,21.0661167286091));
#37348=CARTESIAN_POINT('Ctrl Pts',(34.4476926648849,0.735353817210617,21.0661358844675));
#37349=CARTESIAN_POINT('Ctrl Pts',(34.3018943159103,0.7083223007901,21.0625655773374));
#37350=CARTESIAN_POINT('Ctrl Pts',(34.1776922995948,0.665147105862844,21.0569823906373));
#37351=CARTESIAN_POINT('Ctrl Pts',(34.0351710176682,0.573870276104217,21.0465010716371));
#37352=CARTESIAN_POINT('Ctrl Pts',(33.9243384424563,0.462339732239533,21.0357669569419));
#37353=CARTESIAN_POINT('Ctrl Pts',(33.8485284690001,0.343927579036483,21.0270930625743));
#37354=CARTESIAN_POINT('Ctrl Pts',(33.8140866906283,0.259980124680835,21.0227969523571));
#37355=CARTESIAN_POINT('Ctrl Pts',(33.8008981126124,0.220338324686709,21.0211227123327));
#37356=CARTESIAN_POINT('Ctrl Pts',(33.7948979815476,0.200368717872555,21.0203528356669));
#37357=CARTESIAN_POINT('Ctrl Pts',(33.7903736414347,0.183624806520544,21.0197681873269));
#37358=CARTESIAN_POINT('Ctrl Pts',(33.7874653554772,0.171861616917887,21.0193901307647));
#37359=CARTESIAN_POINT('Ctrl Pts',(33.7858759264221,0.165136687330697,21.019183071464));
#37360=CARTESIAN_POINT('Ctrl Pts',(33.7604707367237,0.0538115303858986,
21.0158657500753));
#37361=CARTESIAN_POINT('Ctrl Pts',(33.7604260304133,-0.0654105160144948,
21.0158728480868));
#37362=CARTESIAN_POINT('Ctrl Pts',(33.7945842900857,-0.200566142677479,
21.0203245347726));
#37363=CARTESIAN_POINT('Ctrl Pts',(33.8113838087165,-0.253576346029871,
21.0224695672281));
#37364=CARTESIAN_POINT('Ctrl Pts',(33.8380574859515,-0.318264908355468,
21.0257877329048));
#37365=CARTESIAN_POINT('Ctrl Pts',(33.8718270287516,-0.379217750812714,
21.0297614242812));
#37366=CARTESIAN_POINT('Ctrl Pts',(33.8986963825208,-0.419278054518851,
21.0327534797157));
#37367=CARTESIAN_POINT('Ctrl Pts',(33.914864910764,-0.4413252762906,21.0345001654573));
#37368=CARTESIAN_POINT('Ctrl Pts',(33.9566653285551,-0.495035919990978,
21.0389217975292));
#37369=CARTESIAN_POINT('Ctrl Pts',(34.0347463980485,-0.573665687092292,
21.0464429283745));
#37370=CARTESIAN_POINT('Ctrl Pts',(34.2243753676715,-0.695811267696493,
21.0605433116086));
#37371=CARTESIAN_POINT('Ctrl Pts',(34.3942976606239,-0.733042633358783,
21.0657866512817));
#37372=CARTESIAN_POINT('Ctrl Pts',(34.5,-0.733042633358783,21.0657866512817));
#37373=CARTESIAN_POINT('Ctrl Pts',(34.5,-0.716521316679393,21.0802569862437));
#37374=CARTESIAN_POINT('Ctrl Pts',(34.6035955276396,-0.716521316679393,
21.0802569862437));
#37375=CARTESIAN_POINT('Ctrl Pts',(34.7700934214207,-0.67988120200932,21.0752351603254));
#37376=CARTESIAN_POINT('Ctrl Pts',(34.9554841655803,-0.560031545890881,
21.06174620078));
#37377=CARTESIAN_POINT('Ctrl Pts',(35.0316640877993,-0.483045905944838,
21.0545626708828));
#37378=CARTESIAN_POINT('Ctrl Pts',(35.0724119772833,-0.430520173076471,
21.0503416889364));
#37379=CARTESIAN_POINT('Ctrl Pts',(35.0881689776849,-0.408964167309974,
21.0486745707798));
#37380=CARTESIAN_POINT('Ctrl Pts',(35.1068677429718,-0.38100104781499,21.0466352576783));
#37381=CARTESIAN_POINT('Ctrl Pts',(35.1274908570911,-0.346013096419943,
21.0443039248873));
#37382=CARTESIAN_POINT('Ctrl Pts',(35.1523989506783,-0.297719928450677,
21.041398164456));
#37383=CARTESIAN_POINT('Ctrl Pts',(35.1731492784692,-0.247200013563418,
21.0388684668766));
#37384=CARTESIAN_POINT('Ctrl Pts',(35.18947918663,-0.195508640474915,21.0368250094389));
#37385=CARTESIAN_POINT('Ctrl Pts',(35.2226686117397,-0.0637516604291672,
21.0325849745592));
#37386=CARTESIAN_POINT('Ctrl Pts',(35.2224214084173,0.0594566848787826,
21.032603908653));
#37387=CARTESIAN_POINT('Ctrl Pts',(35.1926215739719,0.182334230931662,21.0364145961305));
#37388=CARTESIAN_POINT('Ctrl Pts',(35.1826997537462,0.217052061121905,21.0376646556839));
#37389=CARTESIAN_POINT('Ctrl Pts',(35.162102724011,0.276951105850991,21.0402309232163));
#37390=CARTESIAN_POINT('Ctrl Pts',(35.0740849976077,0.458253527328016,21.0506706970671));
#37391=CARTESIAN_POINT('Ctrl Pts',(34.9381177331784,0.585779234560039,21.0644165245667));
#37392=CARTESIAN_POINT('Ctrl Pts',(34.7885727382217,0.655262419714956,21.0726458369329));
#37393=CARTESIAN_POINT('Ctrl Pts',(34.754812924057,0.669293458460397,21.0743424222905));
#37394=CARTESIAN_POINT('Ctrl Pts',(34.6945135464767,0.690607625873672,21.0769736424148));
#37395=CARTESIAN_POINT('Ctrl Pts',(34.5689072989699,0.718490945008162,21.0805729546284));
#37396=CARTESIAN_POINT('Ctrl Pts',(34.4487264809167,0.718795178970658,21.0805912682326));
#37397=CARTESIAN_POINT('Ctrl Pts',(34.3058718218342,0.692218093072797,21.0771713595635));
#37398=CARTESIAN_POINT('Ctrl Pts',(34.184243402737,0.649784071262686,21.0718246698848));
#37399=CARTESIAN_POINT('Ctrl Pts',(34.0449020201095,0.560228358342142,21.0617979579402));
#37400=CARTESIAN_POINT('Ctrl Pts',(33.9367526065258,0.451020124145838,21.0515429755697));
#37401=CARTESIAN_POINT('Ctrl Pts',(33.8629219949076,0.335314040155129,21.0432678615043));
#37402=CARTESIAN_POINT('Ctrl Pts',(33.8294235159375,0.253405458046626,21.0391731603601));
#37403=CARTESIAN_POINT('Ctrl Pts',(33.8166001713389,0.214743037640408,21.0375777885116));
#37404=CARTESIAN_POINT('Ctrl Pts',(33.8107672719337,0.195270124177129,21.0368442715964));
#37405=CARTESIAN_POINT('Ctrl Pts',(33.8063696108869,0.178945108762379,21.0362872895345));
#37406=CARTESIAN_POINT('Ctrl Pts',(33.8035430565577,0.167477411681154,21.0359271500594));
#37407=CARTESIAN_POINT('Ctrl Pts',(33.8019983561009,0.160921727677303,21.0357299093627));
#37408=CARTESIAN_POINT('Ctrl Pts',(33.7773092196027,0.0524018647745844,
21.0325700014518));
#37409=CARTESIAN_POINT('Ctrl Pts',(33.7772644916236,-0.0636976769205621,
21.0325767026177));
#37410=CARTESIAN_POINT('Ctrl Pts',(33.8104612552768,-0.195461551963477,
21.036817273572));
#37411=CARTESIAN_POINT('Ctrl Pts',(33.8267939783758,-0.247157366383319,
21.0388611305665));
#37412=CARTESIAN_POINT('Ctrl Pts',(33.8527381931904,-0.310276045179468,
21.0420238231594));
#37413=CARTESIAN_POINT('Ctrl Pts',(33.8856128252833,-0.369802952328985,
21.0458136904627));
#37414=CARTESIAN_POINT('Ctrl Pts',(33.9117897291869,-0.408954883478312,
21.0486688126864));
#37415=CARTESIAN_POINT('Ctrl Pts',(33.9275474337088,-0.430510250702555,
21.0503359836173));
#37416=CARTESIAN_POINT('Ctrl Pts',(33.9682959366642,-0.483036633717241,
21.0545570798326));
#37417=CARTESIAN_POINT('Ctrl Pts',(34.044487370967,-0.560024633629738,21.0617422024572));
#37418=CARTESIAN_POINT('Ctrl Pts',(34.2298807119576,-0.679875162841163,
21.075231540361));
#37419=CARTESIAN_POINT('Ctrl Pts',(34.3964044723605,-0.716521316679393,
21.0802569862437));
#37420=CARTESIAN_POINT('Ctrl Pts',(34.5,-0.716521316679393,21.0802569862437));
#37421=CARTESIAN_POINT('Ctrl Pts',(34.5,-0.700000000000003,21.0947273212057));
#37422=CARTESIAN_POINT('Ctrl Pts',(34.601488715903,-0.700000000000003,21.0947273212057));
#37423=CARTESIAN_POINT('Ctrl Pts',(34.7645885272708,-0.663944529159921,
21.0899232558818));
#37424=CARTESIAN_POINT('Ctrl Pts',(34.9457436875169,-0.546389858232665,
21.0770453277506));
#37425=CARTESIAN_POINT('Ctrl Pts',(35.0200341754608,-0.47104574396436,21.0701977474631));
#37426=CARTESIAN_POINT('Ctrl Pts',(35.0597301598872,-0.419704240867174,
21.0661772971794));
#37427=CARTESIAN_POINT('Ctrl Pts',(35.0750763502745,-0.398640101910067,
21.064589691873));
#37428=CARTESIAN_POINT('Ctrl Pts',(35.0932804848699,-0.371325740878547,
21.0626481861578));
#37429=CARTESIAN_POINT('Ctrl Pts',(35.1133479175623,-0.337167414446145,
21.0604294914866));
#37430=CARTESIAN_POINT('Ctrl Pts',(35.1375733098774,-0.290042566100743,
21.0576650892507));
#37431=CARTESIAN_POINT('Ctrl Pts',(35.1577401476323,-0.240779148147267,
21.0552597551832));
#37432=CARTESIAN_POINT('Ctrl Pts',(35.1736033280572,-0.190402020471786,
21.0533174556068));
#37433=CARTESIAN_POINT('Ctrl Pts',(35.2058313314997,-0.0620365235102061,
21.0492885267774));
#37434=CARTESIAN_POINT('Ctrl Pts',(35.2055885298052,0.0578604693840868,
21.0493067818511));
#37435=CARTESIAN_POINT('Ctrl Pts',(35.1766521178085,0.177570048832669,21.0529277392257));
#37436=CARTESIAN_POINT('Ctrl Pts',(35.1670153810713,0.211399604550296,21.0541157584863));
#37437=CARTESIAN_POINT('Ctrl Pts',(35.1470037065095,0.269786333607069,21.0565553991735));
#37438=CARTESIAN_POINT('Ctrl Pts',(35.0614301861815,0.446655796342623,21.0664840198707));
#37439=CARTESIAN_POINT('Ctrl Pts',(34.9288635892265,0.571611206123511,21.0795913995426));
#37440=CARTESIAN_POINT('Ctrl Pts',(34.7825768557976,0.639818872896985,21.0874527336103));
#37441=CARTESIAN_POINT('Ctrl Pts',(34.7495454776053,0.653595643122729,21.0890735928326));
#37442=CARTESIAN_POINT('Ctrl Pts',(34.6905269822415,0.67453112887939,21.0915880263274));
#37443=CARTESIAN_POINT('Ctrl Pts',(34.5675200754451,0.701939348923384,21.0950291806477));
#37444=CARTESIAN_POINT('Ctrl Pts',(34.4497602969485,0.7022365407307,21.0950466519978));
#37445=CARTESIAN_POINT('Ctrl Pts',(34.3098493277581,0.676113885355495,21.0917771417895));
#37446=CARTESIAN_POINT('Ctrl Pts',(34.1907945058791,0.634421036662527,21.0866669491324));
#37447=CARTESIAN_POINT('Ctrl Pts',(34.0546330225508,0.546586440580067,21.0770948442432));
#37448=CARTESIAN_POINT('Ctrl Pts',(33.9491667705954,0.439700516052144,21.0673189941975));
#37449=CARTESIAN_POINT('Ctrl Pts',(33.877315520815,0.326700501273774,21.0594426604343));
#37450=CARTESIAN_POINT('Ctrl Pts',(33.8447603412467,0.246830791412416,21.0555493683631));
#37451=CARTESIAN_POINT('Ctrl Pts',(33.8323022300653,0.209147750594108,21.0540328646905));
#37452=CARTESIAN_POINT('Ctrl Pts',(33.8266365623199,0.190171530481702,21.0533357075259));
#37453=CARTESIAN_POINT('Ctrl Pts',(33.8223655803391,0.174265411004215,21.052806391742));
#37454=CARTESIAN_POINT('Ctrl Pts',(33.8196207576382,0.163093206444423,21.052464169354));
#37455=CARTESIAN_POINT('Ctrl Pts',(33.8181207857797,0.156706768023909,21.0522767472613));
#37456=CARTESIAN_POINT('Ctrl Pts',(33.7941477024817,0.050992199163271,21.0492742528283));
#37457=CARTESIAN_POINT('Ctrl Pts',(33.7941029528339,-0.0619848378266299,
21.0492805571486));
#37458=CARTESIAN_POINT('Ctrl Pts',(33.8263382204678,-0.190356961249475,
21.0533100123713));
#37459=CARTESIAN_POINT('Ctrl Pts',(33.8422041480351,-0.240738386736766,
21.0552526939049));
#37460=CARTESIAN_POINT('Ctrl Pts',(33.8674189004292,-0.302287182003468,
21.0582599134139));
#37461=CARTESIAN_POINT('Ctrl Pts',(33.8993986218151,-0.360388153845254,
21.0618659566443));
#37462=CARTESIAN_POINT('Ctrl Pts',(33.9248830758529,-0.398631712437772,
21.064584145657));
#37463=CARTESIAN_POINT('Ctrl Pts',(33.9402299566535,-0.41969522511451,21.0661718017773));
#37464=CARTESIAN_POINT('Ctrl Pts',(33.9799265447732,-0.471037347443503,
21.070192362136));
#37465=CARTESIAN_POINT('Ctrl Pts',(34.0542283438855,-0.546383580167183,
21.07704147654));
#37466=CARTESIAN_POINT('Ctrl Pts',(34.2353860562437,-0.663939057985833,
21.0899197691134));
#37467=CARTESIAN_POINT('Ctrl Pts',(34.398511284097,-0.700000000000003,21.0947273212057));
#37468=CARTESIAN_POINT('Ctrl Pts',(34.5,-0.700000000000003,21.0947273212057));
#37469=CARTESIAN_POINT('',(34.5,-0.749563950038174,21.0513163163198));
#37470=CARTESIAN_POINT('',(34.5,-0.700000000000003,21.0947273212057));
#37471=CARTESIAN_POINT('',(34.5,-0.749563950038172,21.0513163163198));
#37472=CARTESIAN_POINT('',(33.7998534840905,-5.89111502284859E-5,21.049993682322));
#37473=CARTESIAN_POINT('Ctrl Pts',(34.5,-0.700000000000003,21.0947273212057));
#37474=CARTESIAN_POINT('Ctrl Pts',(34.601488715903,-0.700000000000003,21.0947273212057));
#37475=CARTESIAN_POINT('Ctrl Pts',(34.7645885272708,-0.663944529159921,
21.0899232558818));
#37476=CARTESIAN_POINT('Ctrl Pts',(34.9457436875169,-0.546389858232665,
21.0770453277506));
#37477=CARTESIAN_POINT('Ctrl Pts',(35.0200341754608,-0.47104574396436,21.0701977474631));
#37478=CARTESIAN_POINT('Ctrl Pts',(35.0597301598872,-0.419704240867174,
21.0661772971794));
#37479=CARTESIAN_POINT('Ctrl Pts',(35.0750763502745,-0.398640101910067,
21.064589691873));
#37480=CARTESIAN_POINT('Ctrl Pts',(35.0932804848699,-0.371325740878547,
21.0626481861578));
#37481=CARTESIAN_POINT('Ctrl Pts',(35.1133479175623,-0.337167414446145,
21.0604294914866));
#37482=CARTESIAN_POINT('Ctrl Pts',(35.1375733098774,-0.290042566100743,
21.0576650892507));
#37483=CARTESIAN_POINT('Ctrl Pts',(35.1577401476323,-0.240779148147267,
21.0552597551832));
#37484=CARTESIAN_POINT('Ctrl Pts',(35.1736033280572,-0.190402020471786,
21.0533174556068));
#37485=CARTESIAN_POINT('Ctrl Pts',(35.2058313314997,-0.0620365235102061,
21.0492885267774));
#37486=CARTESIAN_POINT('Ctrl Pts',(35.2055885298052,0.0578604693840868,
21.0493067818511));
#37487=CARTESIAN_POINT('Ctrl Pts',(35.1766521178085,0.177570048832669,21.0529277392257));
#37488=CARTESIAN_POINT('Ctrl Pts',(35.1670153810713,0.211399604550296,21.0541157584863));
#37489=CARTESIAN_POINT('Ctrl Pts',(35.1470037065095,0.269786333607069,21.0565553991735));
#37490=CARTESIAN_POINT('Ctrl Pts',(35.0614301861815,0.446655796342623,21.0664840198707));
#37491=CARTESIAN_POINT('Ctrl Pts',(34.9288635892265,0.571611206123511,21.0795913995426));
#37492=CARTESIAN_POINT('Ctrl Pts',(34.7825768557976,0.639818872896985,21.0874527336103));
#37493=CARTESIAN_POINT('Ctrl Pts',(34.7495454776053,0.653595643122729,21.0890735928326));
#37494=CARTESIAN_POINT('Ctrl Pts',(34.6905269822415,0.67453112887939,21.0915880263274));
#37495=CARTESIAN_POINT('Ctrl Pts',(34.5675200754451,0.701939348923384,21.0950291806477));
#37496=CARTESIAN_POINT('Ctrl Pts',(34.4497602969485,0.7022365407307,21.0950466519978));
#37497=CARTESIAN_POINT('Ctrl Pts',(34.3098493277581,0.676113885355495,21.0917771417895));
#37498=CARTESIAN_POINT('Ctrl Pts',(34.1907945058791,0.634421036662527,21.0866669491324));
#37499=CARTESIAN_POINT('Ctrl Pts',(34.0546330225508,0.546586440580067,21.0770948442432));
#37500=CARTESIAN_POINT('Ctrl Pts',(33.9491667705954,0.439700516052144,21.0673189941975));
#37501=CARTESIAN_POINT('Ctrl Pts',(33.877315520815,0.326700501273774,21.0594426604343));
#37502=CARTESIAN_POINT('Ctrl Pts',(33.8447603412467,0.246830791412416,21.0555493683631));
#37503=CARTESIAN_POINT('Ctrl Pts',(33.8323022300653,0.209147750594108,21.0540328646905));
#37504=CARTESIAN_POINT('Ctrl Pts',(33.8266365623199,0.190171530481702,21.0533357075259));
#37505=CARTESIAN_POINT('Ctrl Pts',(33.8223655803391,0.174265411004215,21.052806391742));
#37506=CARTESIAN_POINT('Ctrl Pts',(33.8196207576382,0.163093206444423,21.052464169354));
#37507=CARTESIAN_POINT('Ctrl Pts',(33.8181207857797,0.156706768023909,21.0522767472613));
#37508=CARTESIAN_POINT('Ctrl Pts',(33.8057710155959,0.102247747701762,21.0507300077049));
#37509=CARTESIAN_POINT('Ctrl Pts',(33.7998596786816,0.0502969342747387,
21.0499923790236));
#37510=CARTESIAN_POINT('Ctrl Pts',(33.7998534840905,-5.89111502284807E-5,
21.049993682322));
#37511=CARTESIAN_POINT('Ctrl Pts',(33.7998534840905,-5.89111502284807E-5,
21.049993682322));
#37512=CARTESIAN_POINT('Ctrl Pts',(33.7998472894994,-0.0504147565751959,
21.0499949856204));
#37513=CARTESIAN_POINT('Ctrl Pts',(33.8069970598875,-0.113333687195768,
21.0508923392377));
#37514=CARTESIAN_POINT('Ctrl Pts',(33.8263382204678,-0.190356961249475,
21.0533100123713));
#37515=CARTESIAN_POINT('Ctrl Pts',(33.8422041480351,-0.240738386736766,
21.0552526939049));
#37516=CARTESIAN_POINT('Ctrl Pts',(33.8674189004292,-0.302287182003468,
21.0582599134139));
#37517=CARTESIAN_POINT('Ctrl Pts',(33.8993986218151,-0.360388153845254,
21.0618659566443));
#37518=CARTESIAN_POINT('Ctrl Pts',(33.9248830758529,-0.398631712437772,
21.064584145657));
#37519=CARTESIAN_POINT('Ctrl Pts',(33.9402299566535,-0.41969522511451,21.0661718017773));
#37520=CARTESIAN_POINT('Ctrl Pts',(33.9799265447732,-0.471037347443503,
21.070192362136));
#37521=CARTESIAN_POINT('Ctrl Pts',(34.0542283438855,-0.546383580167183,
21.07704147654));
#37522=CARTESIAN_POINT('Ctrl Pts',(34.2353860562437,-0.663939057985833,
21.0899197691134));
#37523=CARTESIAN_POINT('Ctrl Pts',(34.398511284097,-0.700000000000003,21.0947273212057));
#37524=CARTESIAN_POINT('Ctrl Pts',(34.5,-0.700000000000003,21.0947273212057));
#37525=CARTESIAN_POINT('Ctrl Pts',(34.5,-0.749563950038174,21.0513163163198));
#37526=CARTESIAN_POINT('Ctrl Pts',(34.3921908488873,-0.749563950038174,
21.0513163163198));
#37527=CARTESIAN_POINT('Ctrl Pts',(34.2188700233853,-0.711747372551822,
21.0458550828561));
#37528=CARTESIAN_POINT('Ctrl Pts',(34.02500542513,-0.587306740554846,21.0311436542917));
#37529=CARTESIAN_POINT('Ctrl Pts',(33.945034720446,-0.507035206264715,21.0232865152258));
#37530=CARTESIAN_POINT('Ctrl Pts',(33.9021823878193,-0.452140301878644,
21.0186643472973));
#37531=CARTESIAN_POINT('Ctrl Pts',(33.8856030358547,-0.42960122555939,21.0168381467451));
#37532=CARTESIAN_POINT('Ctrl Pts',(33.8580412322199,-0.388632549296444,
21.0137091580996));
#37533=CARTESIAN_POINT('Ctrl Pts',(33.8233767787127,-0.326253771531467,
21.0095516426503));
#37534=CARTESIAN_POINT('Ctrl Pts',(33.7959736390573,-0.259995325676423,
21.0060780038898));
#37535=CARTESIAN_POINT('Ctrl Pts',(33.7787073248947,-0.20567073339148,21.0038317959733));
#37536=CARTESIAN_POINT('Ctrl Pts',(33.743587569203,-0.0671233551084263,
20.9991689935559));
#37537=CARTESIAN_POINT('Ctrl Pts',(33.7436322538446,0.0552211959972136,
20.9991614986988));
#37538=CARTESIAN_POINT('Ctrl Pts',(33.7697534967433,0.169351646984093,21.0026362335653));
#37539=CARTESIAN_POINT('Ctrl Pts',(33.7713876543967,0.17624582215462,21.00285311147));
#37540=CARTESIAN_POINT('Ctrl Pts',(33.7743776719825,0.188304504278709,21.0032490851194));
#37541=CARTESIAN_POINT('Ctrl Pts',(33.7790286911615,0.205467311567983,21.0038613997373));
#37542=CARTESIAN_POINT('Ctrl Pts',(33.785196053886,0.225933611733011,21.0046676361538));
#37543=CARTESIAN_POINT('Ctrl Pts',(33.7987498653191,0.266554791315046,21.0064207443541));
#37544=CARTESIAN_POINT('Ctrl Pts',(33.8341349430927,0.352541117917839,21.0109182636443));
#37545=CARTESIAN_POINT('Ctrl Pts',(33.9119242783867,0.473659340333228,21.019990938314));
#37546=CARTESIAN_POINT('Ctrl Pts',(34.0254400152268,0.587512193866294,21.0312041853341));
#37547=CARTESIAN_POINT('Ctrl Pts',(34.1711411964527,0.680510140463003,21.0421401113897));
#37548=CARTESIAN_POINT('Ctrl Pts',(34.2979168099864,0.724426508507403,21.0479597951114));
#37549=CARTESIAN_POINT('Ctrl Pts',(34.4466588488531,0.751912455450576,21.0516805007024));
#37550=CARTESIAN_POINT('Ctrl Pts',(34.5716817460195,0.751594137177719,21.0516605025898));
#37551=CARTESIAN_POINT('Ctrl Pts',(34.702486674947,0.722760619862234,21.0477448745898));
#37552=CARTESIAN_POINT('Ctrl Pts',(34.7653478169603,0.700689089135733,21.0448800812064));
#37553=CARTESIAN_POINT('Ctrl Pts',(34.8005645030701,0.686149513350896,21.043032043578));
#37554=CARTESIAN_POINT('Ctrl Pts',(34.9566260210823,0.614115291433095,21.0340667746151));
#37555=CARTESIAN_POINT('Ctrl Pts',(35.0993946204602,0.481448989298802,21.0190440514598));
#37556=CARTESIAN_POINT('Ctrl Pts',(35.1923007590141,0.291280650338835,21.0075819713019));
#37557=CARTESIAN_POINT('Ctrl Pts',(35.214068499096,0.228356974265122,21.004762450079));
#37558=CARTESIAN_POINT('Ctrl Pts',(35.2245604862986,0.191862595129649,21.0033883099402));
#37559=CARTESIAN_POINT('Ctrl Pts',(35.2560871656414,0.0626491158681729,
20.9991981622569));
#37560=CARTESIAN_POINT('Ctrl Pts',(35.2563431722199,-0.0671819342670894,
20.9991778701227));
#37561=CARTESIAN_POINT('Ctrl Pts',(35.2212309037757,-0.205721880481172,
21.0038401171032));
#37562=CARTESIAN_POINT('Ctrl Pts',(35.2039675401431,-0.260041744395718,
21.0060858902635));
#37563=CARTESIAN_POINT('Ctrl Pts',(35.1820502322802,-0.313074653150546,
21.0088643148667));
#37564=CARTESIAN_POINT('Ctrl Pts',(35.1557767361487,-0.363704460367538,
21.0120527916887));
#37565=CARTESIAN_POINT('Ctrl Pts',(35.1340422591755,-0.400351661687876,
21.0146094007192));
#37566=CARTESIAN_POINT('Ctrl Pts',(35.1143542325059,-0.429612298109788,
21.0168443285933));
#37567=CARTESIAN_POINT('Ctrl Pts',(35.0977756120755,-0.452152037495066,
21.0186704724503));
#37568=CARTESIAN_POINT('Ctrl Pts',(35.0549239124764,-0.507046229905794,
21.0232925177222));
#37569=CARTESIAN_POINT('Ctrl Pts',(34.974965121707,-0.587314921207312,21.0311479468387));
#37570=CARTESIAN_POINT('Ctrl Pts',(34.7811032097204,-0.711754547708119,
21.0458589692126));
#37571=CARTESIAN_POINT('Ctrl Pts',(34.6078091511127,-0.749563950038172,
21.0513163163198));
#37572=CARTESIAN_POINT('Ctrl Pts',(34.5,-0.749563950038172,21.0513163163198));
#37573=CARTESIAN_POINT('Origin',(22.,0.,26.5));
#37574=CARTESIAN_POINT('',(35.75,5.5,26.5));
#37575=CARTESIAN_POINT('',(35.75,-5.5,26.5));
#37576=CARTESIAN_POINT('Origin',(35.75,0.,26.5));
#37577=CARTESIAN_POINT('Origin',(35.75,0.,26.5));
#37578=CARTESIAN_POINT('',(22.,-5.5,26.5));
#37579=CARTESIAN_POINT('',(30.8830878247779,3.69831793009931,22.4290732637163));
#37580=CARTESIAN_POINT('',(17.652334347801,3.69831792998691,22.4290732641403));
#37581=CARTESIAN_POINT('',(22.,3.69831792998691,22.4290732641403));
#37582=CARTESIAN_POINT('',(17.5228104013601,3.65742449835961,22.3922943096177));
#37583=CARTESIAN_POINT('Ctrl Pts',(17.652334347801,3.69831792998691,22.4290732641403));
#37584=CARTESIAN_POINT('Ctrl Pts',(17.6306520542537,3.69154163615065,22.4229171992883));
#37585=CARTESIAN_POINT('Ctrl Pts',(17.6089792165843,3.68473366139296,22.4167631015483));
#37586=CARTESIAN_POINT('Ctrl Pts',(17.5873157886876,3.67789386157419,22.410611298869));
#37587=CARTESIAN_POINT('Ctrl Pts',(17.5658049795975,3.67110224813158,22.4045028356273));
#37588=CARTESIAN_POINT('Ctrl Pts',(17.5443035273164,3.66427928145294,22.3983966577005));
#37589=CARTESIAN_POINT('Ctrl Pts',(17.5228113888221,3.65742482201821,22.3922930879342));
#37590=CARTESIAN_POINT('',(17.5228104013601,-3.65742449835961,22.3922943096177));
#37591=CARTESIAN_POINT('Ctrl Pts',(17.5228104013601,3.65742449835962,22.3922943096177));
#37592=CARTESIAN_POINT('Ctrl Pts',(17.4718155231826,3.61371163342318,22.3533731903452));
#37593=CARTESIAN_POINT('Ctrl Pts',(17.4213621793917,3.56860095253652,22.314462944171));
#37594=CARTESIAN_POINT('Ctrl Pts',(17.1786673062269,3.34189405579382,22.1254229108229));
#37595=CARTESIAN_POINT('Ctrl Pts',(16.9998567608571,3.14235547380069,21.9800060560567));
#37596=CARTESIAN_POINT('Ctrl Pts',(16.7079762629281,2.75740413257784,21.7359762518195));
#37597=CARTESIAN_POINT('Ctrl Pts',(16.5729905746261,2.54826816026991,21.6195359147249));
#37598=CARTESIAN_POINT('Ctrl Pts',(16.333784841218,2.09462553853969,21.4083259944966));
#37599=CARTESIAN_POINT('Ctrl Pts',(16.2295518424091,1.85008857261991,21.3136362055264));
#37600=CARTESIAN_POINT('Ctrl Pts',(16.061681316055,1.33934953012783,21.1589004443208));
#37601=CARTESIAN_POINT('Ctrl Pts',(15.9978650437258,1.07266052861995,21.098765657674));
#37602=CARTESIAN_POINT('Ctrl Pts',(15.9139403163524,0.53468492332373,21.0193025010528));
#37603=CARTESIAN_POINT('Ctrl Pts',(15.8938293331417,0.263394893211526,21.));
#37604=CARTESIAN_POINT('Ctrl Pts',(15.8938293331417,0.,21.));
#37605=CARTESIAN_POINT('Ctrl Pts',(15.8938293331417,-0.263394893211527,
21.));
#37606=CARTESIAN_POINT('Ctrl Pts',(15.9139403163524,-0.534684923323731,
21.0193025010528));
#37607=CARTESIAN_POINT('Ctrl Pts',(15.9978650437258,-1.07266052861995,21.098765657674));
#37608=CARTESIAN_POINT('Ctrl Pts',(16.061681316055,-1.33934953012783,21.1589004443208));
#37609=CARTESIAN_POINT('Ctrl Pts',(16.2295518424091,-1.85008857261992,21.3136362055264));
#37610=CARTESIAN_POINT('Ctrl Pts',(16.333784841218,-2.09462553853969,21.4083259944966));
#37611=CARTESIAN_POINT('Ctrl Pts',(16.5729905746261,-2.5482681602699,21.6195359147249));
#37612=CARTESIAN_POINT('Ctrl Pts',(16.7079762629281,-2.75740413257784,21.7359762518195));
#37613=CARTESIAN_POINT('Ctrl Pts',(16.9998567608571,-3.14235547380069,21.9800060560567));
#37614=CARTESIAN_POINT('Ctrl Pts',(17.1786673062269,-3.34189405579382,22.1254229108229));
#37615=CARTESIAN_POINT('Ctrl Pts',(17.4213621793917,-3.56860095253652,22.314462944171));
#37616=CARTESIAN_POINT('Ctrl Pts',(17.4718155231826,-3.61371163342317,22.3533731903451));
#37617=CARTESIAN_POINT('Ctrl Pts',(17.5228104013601,-3.65742449835961,22.3922943096177));
#37618=CARTESIAN_POINT('',(17.652334347801,-3.69831792998691,22.4290732641403));
#37619=CARTESIAN_POINT('Ctrl Pts',(17.5228110788605,-3.65742469016367,22.3922935859358));
#37620=CARTESIAN_POINT('Ctrl Pts',(17.5443017343427,-3.66427868717436,22.3983965430443));
#37621=CARTESIAN_POINT('Ctrl Pts',(17.5658016777307,-3.67110118593092,22.4045021463312));
#37622=CARTESIAN_POINT('Ctrl Pts',(17.5873109511853,-3.67789232535356,22.4106100751017));
#37623=CARTESIAN_POINT('Ctrl Pts',(17.6089760162179,-3.68473265297072,22.4167622435748));
#37624=CARTESIAN_POINT('Ctrl Pts',(17.6306504666714,-3.69154113998894,22.4229167485399));
#37625=CARTESIAN_POINT('Ctrl Pts',(17.652334347801,-3.69831792998691,22.4290732641403));
#37626=CARTESIAN_POINT('',(30.8830878255874,-3.69831792998913,22.4290732641319));
#37627=CARTESIAN_POINT('',(22.,-3.69831792998691,22.4290732641403));
#37628=CARTESIAN_POINT('',(31.3,-3.55458559184835,22.3029866249648));
#37629=CARTESIAN_POINT('Ctrl Pts',(30.8830878256038,-3.69831792998691,22.4290732641403));
#37630=CARTESIAN_POINT('Ctrl Pts',(30.9233724031233,-3.69831792998691,22.4290732641403));
#37631=CARTESIAN_POINT('Ctrl Pts',(30.9634974147365,-3.69473776211815,22.4258129546819));
#37632=CARTESIAN_POINT('Ctrl Pts',(31.0608268115351,-3.67754139921518,22.4102713040562));
#37633=CARTESIAN_POINT('Ctrl Pts',(31.1158542155423,-3.66015163820752,22.3946036369474));
#37634=CARTESIAN_POINT('Ctrl Pts',(31.2213217785344,-3.61140543651387,22.3516419451064));
#37635=CARTESIAN_POINT('Ctrl Pts',(31.2646787460225,-3.58223402584168,22.3264096749149));
#37636=CARTESIAN_POINT('Ctrl Pts',(31.2994908266689,-3.55498492904841,22.3033248609664));
#37637=CARTESIAN_POINT('Ctrl Pts',(31.2997454942081,-3.55478532723142,22.3031557872837));
#37638=CARTESIAN_POINT('Ctrl Pts',(31.3,-3.55458559184835,22.3029866249648));
#37639=CARTESIAN_POINT('',(31.3,3.55458559184835,22.3029866249648));
#37640=CARTESIAN_POINT('Origin',(31.3,0.,26.5));
#37641=CARTESIAN_POINT('Ctrl Pts',(31.3,3.55458559184835,22.3029866249648));
#37642=CARTESIAN_POINT('Ctrl Pts',(31.2997454945137,3.55478532699163,22.3031557870806));
#37643=CARTESIAN_POINT('Ctrl Pts',(31.2994908263624,3.55498492928751,22.3033248611689));
#37644=CARTESIAN_POINT('Ctrl Pts',(31.266221424283,3.58102649708782,22.3253866840674));
#37645=CARTESIAN_POINT('Ctrl Pts',(31.2312555016837,3.60401240458897,22.3452673820714));
#37646=CARTESIAN_POINT('Ctrl Pts',(31.1529671626145,3.64446341500391,22.3807010381468));
#37647=CARTESIAN_POINT('Ctrl Pts',(31.1107407752369,3.66112199589451,22.3955556214492));
#37648=CARTESIAN_POINT('Ctrl Pts',(31.007251686649,3.68975720344199,22.421254208944));
#37649=CARTESIAN_POINT('Ctrl Pts',(30.9454996143513,3.69831792998691,22.4290732641403));
#37650=CARTESIAN_POINT('Ctrl Pts',(30.8830878256038,3.69831792998691,22.4290732641403));
#37651=CARTESIAN_POINT('Origin',(34.5,0.,20.6));
#37652=CARTESIAN_POINT('',(33.8,-8.57252759403151E-17,21.2));
#37653=CARTESIAN_POINT('',(33.8,-8.57252759403151E-17,20.6));
#37654=CARTESIAN_POINT('Origin',(34.5,0.,21.2));
#37655=CARTESIAN_POINT('Origin',(35.7926776695297,0.,26.5));
#37656=CARTESIAN_POINT('',(35.7926776695297,5.48232233047034,26.5));
#37657=CARTESIAN_POINT('Origin',(10.025,4.525,14.25));
#37658=CARTESIAN_POINT('',(10.05,4.5,8.95830089865303));
#37659=CARTESIAN_POINT('',(10.,4.55,8.96086067249887));
#37660=CARTESIAN_POINT('',(10.025,4.525,8.95958078557592));
#37661=CARTESIAN_POINT('',(10.,4.55,6.2));
#37662=CARTESIAN_POINT('',(10.,4.55,14.25));
#37663=CARTESIAN_POINT('',(10.05,4.5,6.2));
#37664=CARTESIAN_POINT('',(13.65,0.900000000000021,6.2));
#37665=CARTESIAN_POINT('',(10.05,4.5,14.25));
#37666=CARTESIAN_POINT('Origin',(10.,0.,14.5));
#37667=CARTESIAN_POINT('',(10.,7.21647899346606,8.96086067249887));
#37668=CARTESIAN_POINT('',(10.,0.,8.96086067249887));
#37669=CARTESIAN_POINT('',(10.,7.94827338858625,6.2));
#37670=CARTESIAN_POINT('',(10.,6.66129870798463,11.0554044768152));
#37671=CARTESIAN_POINT('',(10.,8.,6.2));
#37672=CARTESIAN_POINT('Origin',(29.2841674687199,4.525,6.98243503368624));
#37673=CARTESIAN_POINT('',(11.2601630224385,4.5,13.9818998597663));
#37674=CARTESIAN_POINT('Origin',(29.2841674687199,4.5,6.98243503368624));
#37675=CARTESIAN_POINT('',(11.2135541721682,4.55,14.));
#37676=CARTESIAN_POINT('',(11.2601630224385,4.5,13.9818998597663));
#37677=CARTESIAN_POINT('Origin',(29.2841674687199,4.55,6.98243503368624));
#37678=CARTESIAN_POINT('Ctrl Pts',(30.9997093954044,-10.0241065289954,4.54380411865086));
#37679=CARTESIAN_POINT('Ctrl Pts',(30.999717504114,-10.0237702568947,4.54398835593614));
#37680=CARTESIAN_POINT('Ctrl Pts',(30.9997551851855,-10.0224440653027,4.54471502897839));
#37681=CARTESIAN_POINT('Ctrl Pts',(30.9998913604463,-10.0153494937356,4.54860165528609));
#37682=CARTESIAN_POINT('Ctrl Pts',(30.999969789191,-10.0087553611579,4.5522132400076));
#37683=CARTESIAN_POINT('Ctrl Pts',(31.0000056927207,-10.001666156019,4.55609602391547));
#37684=CARTESIAN_POINT('Ctrl Pts',(31.,-10.0003364131356,4.55682446904928));
#37685=CARTESIAN_POINT('Ctrl Pts',(31.,-10.,4.55700877125496));
#37686=CARTESIAN_POINT('Ctrl Pts',(30.9987342290661,-10.0081103673502,4.51459940199573));
#37687=CARTESIAN_POINT('Ctrl Pts',(30.9987548546594,-10.0075127982384,4.51492503645021));
#37688=CARTESIAN_POINT('Ctrl Pts',(30.998879062242,-10.0045941559398,4.51651823692996));
#37689=CARTESIAN_POINT('Ctrl Pts',(30.9992674697787,-9.99306598674585,4.522824317168));
#37690=CARTESIAN_POINT('Ctrl Pts',(30.9996846757043,-9.98035171628815,4.52977717483027));
#37691=CARTESIAN_POINT('Ctrl Pts',(30.9999513534079,-9.96882779683825,4.53608128171654));
#37692=CARTESIAN_POINT('Ctrl Pts',(31.,-9.96590392822198,4.53767905786143));
#37693=CARTESIAN_POINT('Ctrl Pts',(31.,-9.96530556667556,4.53800584750331));
#37694=CARTESIAN_POINT('Ctrl Pts',(30.9977590627279,-9.99211420570491,4.4853946853406));
#37695=CARTESIAN_POINT('Ctrl Pts',(30.9978068742384,-9.99125477325143,4.48586153734842));
#37696=CARTESIAN_POINT('Ctrl Pts',(30.9981151602182,-9.98842961893862,4.48739695061579));
#37697=CARTESIAN_POINT('Ctrl Pts',(30.9989671002748,-9.96926330090421,4.49792896802917));
#37698=CARTESIAN_POINT('Ctrl Pts',(30.9997226844942,-9.95345281891056,4.50656389269967));
#37699=CARTESIAN_POINT('Ctrl Pts',(30.9999327268108,-9.93430937953765,4.51701465622552));
#37700=CARTESIAN_POINT('Ctrl Pts',(31.,-9.9314714433084,4.51853364667358));
#37701=CARTESIAN_POINT('Ctrl Pts',(31.,-9.93061113335113,4.51900292375165));
#37702=CARTESIAN_POINT('Ctrl Pts',(30.9967838963896,-9.97611804405966,4.45618996868547));
#37703=CARTESIAN_POINT('Ctrl Pts',(30.9968734777971,-9.97499807737716,4.4567968232885));
#37704=CARTESIAN_POINT('Ctrl Pts',(30.9972889013038,-9.97058210687397,4.45918088219282));
#37705=CARTESIAN_POINT('Ctrl Pts',(30.9987939241305,-9.94698231574099,4.47201457241229));
#37706=CARTESIAN_POINT('Ctrl Pts',(30.9996655003134,-9.92505068401682,4.48403716442464));
#37707=CARTESIAN_POINT('Ctrl Pts',(31.0000630457773,-9.9014713472524,4.4969678159358));
#37708=CARTESIAN_POINT('Ctrl Pts',(31.,-9.89703895839481,4.49938823548573));
#37709=CARTESIAN_POINT('Ctrl Pts',(31.,-9.89591670002669,4.5));
#37710=CARTESIAN_POINT('',(31.,-10.,4.55700877125496));
#37711=CARTESIAN_POINT('',(30.9997093954044,-10.0241065289954,4.54380411865086));
#37712=CARTESIAN_POINT('Ctrl Pts',(31.,-10.,4.55700877125496));
#37713=CARTESIAN_POINT('Ctrl Pts',(31.,-10.0001511977844,4.55692593832657));
#37714=CARTESIAN_POINT('Ctrl Pts',(30.99999997723,-10.0003064755069,4.55684087080203));
#37715=CARTESIAN_POINT('Ctrl Pts',(30.9999998614271,-10.0005264462905,4.55672037207584));
#37716=CARTESIAN_POINT('Ctrl Pts',(30.9999997332039,-10.0007700100071,4.55658694927716));
#37717=CARTESIAN_POINT('Ctrl Pts',(30.9999994933958,-10.0010926664444,4.55641020889953));
#37718=CARTESIAN_POINT('Ctrl Pts',(30.9999988481894,-10.0015177680866,4.55617736226788));
#37719=CARTESIAN_POINT('Ctrl Pts',(30.9999981092284,-10.0020046409568,4.55591068085195));
#37720=CARTESIAN_POINT('Ctrl Pts',(30.9999968155925,-10.0026250944535,4.55557084135448));
#37721=CARTESIAN_POINT('Ctrl Pts',(30.9999943960859,-10.0033478047717,4.55517500045817));
#37722=CARTESIAN_POINT('Ctrl Pts',(30.9999912612891,-10.0042841733556,4.55466213524763));
#37723=CARTESIAN_POINT('Ctrl Pts',(30.9999861247383,-10.0053881015756,4.55405750553938));
#37724=CARTESIAN_POINT('Ctrl Pts',(30.9999787444039,-10.0065200261086,4.55343754627602));
#37725=CARTESIAN_POINT('Ctrl Pts',(30.9999728171858,-10.0074290856682,4.55293965098492));
#37726=CARTESIAN_POINT('Ctrl Pts',(30.9999655114504,-10.0083524798443,4.55243390713277));
#37727=CARTESIAN_POINT('Ctrl Pts',(30.9999573089849,-10.0092401411061,4.55194773309642));
#37728=CARTESIAN_POINT('Ctrl Pts',(30.9999505385552,-10.0099728291229,4.55154643824915));
#37729=CARTESIAN_POINT('Ctrl Pts',(30.9999431979467,-10.0106807421438,4.55115871205554));
#37730=CARTESIAN_POINT('Ctrl Pts',(30.9999353410503,-10.011371619,4.55078031184829));
#37731=CARTESIAN_POINT('Ctrl Pts',(30.9999270910272,-10.0120970644781,4.55038297805887));
#37732=CARTESIAN_POINT('Ctrl Pts',(30.9999182331629,-10.0128091740849,4.54999294271822));
#37733=CARTESIAN_POINT('Ctrl Pts',(30.9999082034238,-10.0135493441069,4.54958752483879));
#37734=CARTESIAN_POINT('Ctrl Pts',(30.9998975941431,-10.0143322828788,4.54915868096885));
#37735=CARTESIAN_POINT('Ctrl Pts',(30.9998856313636,-10.0151465414471,4.54871266747929));
#37736=CARTESIAN_POINT('Ctrl Pts',(30.9998723241665,-10.0159792166846,4.54825654888553));
#37737=CARTESIAN_POINT('Ctrl Pts',(30.9998546050825,-10.017087958249,4.54764920808756));
#37738=CARTESIAN_POINT('Ctrl Pts',(30.9998344176981,-10.0182272517748,4.54702510047069));
#37739=CARTESIAN_POINT('Ctrl Pts',(30.9998142444384,-10.0192737287039,4.5464518136809));
#37740=CARTESIAN_POINT('Ctrl Pts',(30.9997977964192,-10.0201269607973,4.54598439134776));
#37741=CARTESIAN_POINT('Ctrl Pts',(30.9997814904077,-10.0209142598129,4.5455530719156));
#37742=CARTESIAN_POINT('Ctrl Pts',(30.9997672645524,-10.0215735191706,4.54519189035887));
#37743=CARTESIAN_POINT('Ctrl Pts',(30.9997549602234,-10.0221437305145,4.54487949460983));
#37744=CARTESIAN_POINT('Ctrl Pts',(30.9997442695991,-10.0226170579556,4.54462017075191));
#37745=CARTESIAN_POINT('Ctrl Pts',(30.9997357958304,-10.0229856158381,4.54441824588489));
#37746=CARTESIAN_POINT('Ctrl Pts',(30.9997282313378,-10.0233146256855,4.54423798852821));
#37747=CARTESIAN_POINT('Ctrl Pts',(30.9997224473027,-10.0235598209633,4.54410364991749));
#37748=CARTESIAN_POINT('Ctrl Pts',(30.9997178906574,-10.023751612567,4.54399857074021));
#37749=CARTESIAN_POINT('Ctrl Pts',(30.999714655592,-10.0238877781751,4.54392396804753));
#37750=CARTESIAN_POINT('Ctrl Pts',(30.9997120192429,-10.0239977171451,4.54386373465786));
#37751=CARTESIAN_POINT('Ctrl Pts',(30.9997093954044,-10.0241065289954,4.54380411865086));
#37752=CARTESIAN_POINT('',(30.9967838963896,-9.97611804405966,4.45618996868547));
#37753=CARTESIAN_POINT('Ctrl Pts',(30.9967838963896,-9.97611804405966,4.45618996868547));
#37754=CARTESIAN_POINT('Ctrl Pts',(30.9977590627279,-9.99211420570491,4.4853946853406));
#37755=CARTESIAN_POINT('Ctrl Pts',(30.9987342290661,-10.0081103673502,4.51459940199573));
#37756=CARTESIAN_POINT('Ctrl Pts',(30.9997093954044,-10.0241065289954,4.54380411865086));
#37757=CARTESIAN_POINT('',(31.,-9.89591670002669,4.5));
#37758=CARTESIAN_POINT('Ctrl Pts',(30.9967838963896,-9.97611804405966,4.45618996868547));
#37759=CARTESIAN_POINT('Ctrl Pts',(30.9968133695279,-9.9757495643299,4.45638962964291));
#37760=CARTESIAN_POINT('Ctrl Pts',(30.996842996836,-9.97537708361651,4.45659147843499));
#37761=CARTESIAN_POINT('Ctrl Pts',(30.9968795362938,-9.97491323183949,4.45684283454683));
#37762=CARTESIAN_POINT('Ctrl Pts',(30.9969179534944,-9.97442554297466,4.45710710771105));
#37763=CARTESIAN_POINT('Ctrl Pts',(30.9969639966797,-9.9738371180411,4.4574259622937));
#37764=CARTESIAN_POINT('Ctrl Pts',(30.9970209278329,-9.97309735320343,4.45782692293292));
#37765=CARTESIAN_POINT('Ctrl Pts',(30.9970817698807,-9.97230677010212,4.45825542762726));
#37766=CARTESIAN_POINT('Ctrl Pts',(30.9971550088046,-9.97134371278461,4.45877750747389));
#37767=CARTESIAN_POINT('Ctrl Pts',(30.9972398674313,-9.97019833928475,4.45939875359796));
#37768=CARTESIAN_POINT('Ctrl Pts',(30.9973345740799,-9.96892004278472,4.46009209663946));
#37769=CARTESIAN_POINT('Ctrl Pts',(30.997443648044,-9.96741519981467,4.46090867672731));
#37770=CARTESIAN_POINT('Ctrl Pts',(30.9975613300434,-9.96572608185513,4.46182599231399));
#37771=CARTESIAN_POINT('Ctrl Pts',(30.9977185936927,-9.96346883898112,4.46305184161574));
#37772=CARTESIAN_POINT('Ctrl Pts',(30.9978907754155,-9.96088399058384,4.46445683844123));
#37773=CARTESIAN_POINT('Ctrl Pts',(30.9980603292894,-9.95815761335659,4.46594063852779));
#37774=CARTESIAN_POINT('Ctrl Pts',(30.9982118909916,-9.95572054504439,4.4672669854971));
#37775=CARTESIAN_POINT('Ctrl Pts',(30.9983610413697,-9.95317546940992,4.46865353040875));
#37776=CARTESIAN_POINT('Ctrl Pts',(30.9984991867338,-9.95065274965857,4.4700294224399));
#37777=CARTESIAN_POINT('Ctrl Pts',(30.9986110688123,-9.94860963274859,4.47114373895232));
#37778=CARTESIAN_POINT('Ctrl Pts',(30.9987158226638,-9.94658204035722,4.47225058167765));
#37779=CARTESIAN_POINT('Ctrl Pts',(30.9988121054087,-9.94460762878096,4.47332931082265));
#37780=CARTESIAN_POINT('Ctrl Pts',(30.9988996657651,-9.9428120819124,4.47431031638482));
#37781=CARTESIAN_POINT('Ctrl Pts',(30.9989802761463,-9.9410609811228,4.47526781120672));
#37782=CARTESIAN_POINT('Ctrl Pts',(30.9990549592769,-9.9393454541988,4.47620648550759));
#37783=CARTESIAN_POINT('Ctrl Pts',(30.9991510543234,-9.93713807967809,4.47741428102861));
#37784=CARTESIAN_POINT('Ctrl Pts',(30.9992376098028,-9.93498836525396,4.47859157980782));
#37785=CARTESIAN_POINT('Ctrl Pts',(30.9993191787092,-9.93278231342343,4.47980026592178));
#37786=CARTESIAN_POINT('Ctrl Pts',(30.9993838570363,-9.9310330716113,4.48075866783194));
#37787=CARTESIAN_POINT('Ctrl Pts',(30.9994453083827,-9.92924717485037,4.48173748465682));
#37788=CARTESIAN_POINT('Ctrl Pts',(30.9995031846701,-9.92741489589081,4.48274188966046));
#37789=CARTESIAN_POINT('Ctrl Pts',(30.9995676886674,-9.92537279328657,4.48386131422348));
#37790=CARTESIAN_POINT('Ctrl Pts',(30.9996276231467,-9.92327363571715,4.4850122227893));
#37791=CARTESIAN_POINT('Ctrl Pts',(30.9996811029328,-9.92115993228124,4.48617116978916));
#37792=CARTESIAN_POINT('Ctrl Pts',(30.9997557460711,-9.91820978103073,4.4877887424736));
#37793=CARTESIAN_POINT('Ctrl Pts',(30.9998173334517,-9.91523262517508,4.48942124714919));
#37794=CARTESIAN_POINT('Ctrl Pts',(30.9998635065226,-9.91244178079622,4.49095138375327));
#37795=CARTESIAN_POINT('Ctrl Pts',(30.9999017819863,-9.91012829242206,4.49221980031967));
#37796=CARTESIAN_POINT('Ctrl Pts',(30.999929592725,-9.90794763352294,4.49341523424628));
#37797=CARTESIAN_POINT('Ctrl Pts',(30.9999490870108,-9.90601712246641,4.49447322866645));
#37798=CARTESIAN_POINT('Ctrl Pts',(30.999964960073,-9.90444521968738,4.49533469193735));
#37799=CARTESIAN_POINT('Ctrl Pts',(30.9999754346307,-9.90303987951068,4.49610464213462));
#37800=CARTESIAN_POINT('Ctrl Pts',(30.9999825498663,-9.90183534326441,4.49676429672001));
#37801=CARTESIAN_POINT('Ctrl Pts',(30.9999891823826,-9.90071252641856,4.49737919833315));
#37802=CARTESIAN_POINT('Ctrl Pts',(30.9999929401154,-9.89976477990244,4.4978979409434));
#37803=CARTESIAN_POINT('Ctrl Pts',(30.9999953264449,-9.89898318387141,4.49832545193876));
#37804=CARTESIAN_POINT('Ctrl Pts',(30.9999975693351,-9.89824856861423,4.49872726577523));
#37805=CARTESIAN_POINT('Ctrl Pts',(30.9999986085518,-9.89766105451709,4.4990483091807));
#37806=CARTESIAN_POINT('Ctrl Pts',(30.9999992167745,-9.89717349943034,4.49931448218875));
#37807=CARTESIAN_POINT('Ctrl Pts',(30.9999998249972,-9.89668594434359,4.49958065519681));
#37808=CARTESIAN_POINT('Ctrl Pts',(31.,-9.89629902896181,4.49979158518045));
#37809=CARTESIAN_POINT('Ctrl Pts',(31.,-9.89591670002669,4.5));
#37810=CARTESIAN_POINT('',(31.,-9.94795835001334,4.52850438562748));
#37811=CARTESIAN_POINT('Ctrl Pts',(30.9967839065843,9.97611791660417,4.45619003774767));
#37812=CARTESIAN_POINT('Ctrl Pts',(30.996873500376,9.97499779333315,4.45679697722312));
#37813=CARTESIAN_POINT('Ctrl Pts',(30.9972889684913,9.97058139404403,4.45918135074556));
#37814=CARTESIAN_POINT('Ctrl Pts',(30.9987938829419,9.94698237497655,4.47201437960008));
#37815=CARTESIAN_POINT('Ctrl Pts',(30.9996653875363,9.92505089721926,4.48403521866371));
#37816=CARTESIAN_POINT('Ctrl Pts',(31.0000630537281,9.90147103509372,4.49696656564785));
#37817=CARTESIAN_POINT('Ctrl Pts',(31.,9.89703887496921,4.49938794717922));
#37818=CARTESIAN_POINT('Ctrl Pts',(31.,9.89591670002669,4.5));
#37819=CARTESIAN_POINT('Ctrl Pts',(30.9977590705465,9.99211407834309,4.4853947546077));
#37820=CARTESIAN_POINT('Ctrl Pts',(30.9978068875849,9.99125454012803,4.48586166403795));
#37821=CARTESIAN_POINT('Ctrl Pts',(30.998073130725,9.98842907687459,4.48738248206113));
#37822=CARTESIAN_POINT('Ctrl Pts',(30.999321036897,9.96926357875824,4.49779643372825));
#37823=CARTESIAN_POINT('Ctrl Pts',(30.9998925790727,9.95345321712367,4.506474317633));
#37824=CARTESIAN_POINT('Ctrl Pts',(31.000104853691,9.93430916936581,4.51698220500682));
#37825=CARTESIAN_POINT('Ctrl Pts',(31.,9.93147138540036,4.51853345740689));
#37826=CARTESIAN_POINT('Ctrl Pts',(31.,9.93061113335113,4.51900292375165));
#37827=CARTESIAN_POINT('Ctrl Pts',(30.9987342345088,10.008110240082,4.51459947146774));
#37828=CARTESIAN_POINT('Ctrl Pts',(30.9987548614373,10.0075126162853,4.51492513567012));
#37829=CARTESIAN_POINT('Ctrl Pts',(30.9989180237843,10.0045936571128,4.51651835890182));
#37830=CARTESIAN_POINT('Ctrl Pts',(30.9993345094708,9.9930603747469,4.52282419804882));
#37831=CARTESIAN_POINT('Ctrl Pts',(30.9997836591977,9.98034689548292,4.5297768367585));
#37832=CARTESIAN_POINT('Ctrl Pts',(30.9999536037935,9.96882556865815,4.53608101051986));
#37833=CARTESIAN_POINT('Ctrl Pts',(31.,9.96590389583151,4.53767896763457));
#37834=CARTESIAN_POINT('Ctrl Pts',(31.,9.96530556667556,4.5380058475033));
#37835=CARTESIAN_POINT('Ctrl Pts',(30.999709398471,10.0241064018209,4.54380418832777));
#37836=CARTESIAN_POINT('Ctrl Pts',(30.9997175072273,10.0237701260067,4.54398842764829));
#37837=CARTESIAN_POINT('Ctrl Pts',(30.9997551883338,10.0224439201123,4.54471510649137));
#37838=CARTESIAN_POINT('Ctrl Pts',(30.9998913599888,10.0153494914902,4.54860164074375));
#37839=CARTESIAN_POINT('Ctrl Pts',(30.9999697880435,10.0087555013957,4.55221317457904));
#37840=CARTESIAN_POINT('Ctrl Pts',(31.0000056930925,10.0016661430369,4.55609605212253));
#37841=CARTESIAN_POINT('Ctrl Pts',(31.,10.0003364062627,4.55682447786224));
#37842=CARTESIAN_POINT('Ctrl Pts',(31.,10.,4.55700877125496));
#37843=CARTESIAN_POINT('',(31.,9.89591670002669,4.5));
#37844=CARTESIAN_POINT('',(30.9967839065843,9.97611791660417,4.45619003774767));
#37845=CARTESIAN_POINT('Ctrl Pts',(31.,9.89591670002669,4.5));
#37846=CARTESIAN_POINT('Ctrl Pts',(31.,9.8962858594512,4.49979865432873));
#37847=CARTESIAN_POINT('Ctrl Pts',(30.9999998340188,9.89665901681545,4.49959511613558));
#37848=CARTESIAN_POINT('Ctrl Pts',(30.9999992772054,9.89712348211803,4.49934145900802));
#37849=CARTESIAN_POINT('Ctrl Pts',(30.9999986917831,9.89761181151393,4.49907476905039));
#37850=CARTESIAN_POINT('Ctrl Pts',(30.9999976809336,9.89820080553401,4.49875282346015));
#37851=CARTESIAN_POINT('Ctrl Pts',(30.9999954505896,9.89894103516699,4.4983478421473));
#37852=CARTESIAN_POINT('Ctrl Pts',(30.9999930670703,9.89973210217239,4.49791504759257));
#37853=CARTESIAN_POINT('Ctrl Pts',(30.9999892819254,9.90069551898937,4.49738762293931));
#37854=CARTESIAN_POINT('Ctrl Pts',(30.9999825049737,9.90184112663191,4.49676013739004));
#37855=CARTESIAN_POINT('Ctrl Pts',(30.999974941968,9.90311961249728,4.49605987023428));
#37856=CARTESIAN_POINT('Ctrl Pts',(30.9999635890354,9.90462446354965,4.49523527848236));
#37857=CARTESIAN_POINT('Ctrl Pts',(30.9999460260694,9.90631345761313,4.49430953032038));
#37858=CARTESIAN_POINT('Ctrl Pts',(30.9999225661086,9.90856955346075,4.49307295013971));
#37859=CARTESIAN_POINT('Ctrl Pts',(30.9998876845076,9.91115273554961,4.4916566847344));
#37860=CARTESIAN_POINT('Ctrl Pts',(30.9998386709666,9.91387735661048,4.49016275480571));
#37861=CARTESIAN_POINT('Ctrl Pts',(30.9997948164941,9.91631518943797,4.4888260729917));
#37862=CARTESIAN_POINT('Ctrl Pts',(30.9997397438994,9.91886117398248,4.48743000956264));
#37863=CARTESIAN_POINT('Ctrl Pts',(30.9996753159154,9.92138482445032,4.48604632553787));
#37864=CARTESIAN_POINT('Ctrl Pts',(30.9996231515921,9.9234281061253,4.48492602134052));
#37865=CARTESIAN_POINT('Ctrl Pts',(30.9995650155982,9.9254558861659,4.48381430249766));
#37866=CARTESIAN_POINT('Ctrl Pts',(30.9995026119473,9.9274304796577,4.48273195330263));
#37867=CARTESIAN_POINT('Ctrl Pts',(30.9994458642117,9.92922610712186,4.48174770213982));
#37868=CARTESIAN_POINT('Ctrl Pts',(30.9993856809681,9.93097728810924,4.48078798814601));
#37869=CARTESIAN_POINT('Ctrl Pts',(30.9993224038945,9.93269285298828,4.47984811356608));
#37870=CARTESIAN_POINT('Ctrl Pts',(30.9992409740201,9.93490057569886,4.47863860964085));
#37871=CARTESIAN_POINT('Ctrl Pts',(30.9991545968578,9.93705051945132,4.47746129227476));
#37872=CARTESIAN_POINT('Ctrl Pts',(30.9990587546962,9.93925671489986,4.47625423743952));
#37873=CARTESIAN_POINT('Ctrl Pts',(30.9989827667415,9.94100588537807,4.47529723035079));
#37874=CARTESIAN_POINT('Ctrl Pts',(30.9989006378005,9.94279166942895,4.47432085377575));
#37875=CARTESIAN_POINT('Ctrl Pts',(30.998811268279,9.94462383248334,4.47331993348054));
#37876=CARTESIAN_POINT('Ctrl Pts',(30.9987116713683,9.94666566707282,4.47220446852495));
#37877=CARTESIAN_POINT('Ctrl Pts',(30.9986029986771,9.9487645445695,4.47105883546725));
#37878=CARTESIAN_POINT('Ctrl Pts',(30.9984867998044,9.95087798782649,4.46990630726323));
#37879=CARTESIAN_POINT('Ctrl Pts',(30.9983246182708,9.95382777090777,4.46829769620369));
#37880=CARTESIAN_POINT('Ctrl Pts',(30.9981474066052,9.95680460084669,4.46667643445956));
#37881=CARTESIAN_POINT('Ctrl Pts',(30.9979698970121,9.95959518572774,4.4651583514365));
#37882=CARTESIAN_POINT('Ctrl Pts',(30.997822707114,9.96190912210162,4.46389956602938));
#37883=CARTESIAN_POINT('Ctrl Pts',(30.9976758219154,9.96409019555147,4.46271431184688));
#37884=CARTESIAN_POINT('Ctrl Pts',(30.9975407431566,9.96602096117105,4.46166586166561));
#37885=CARTESIAN_POINT('Ctrl Pts',(30.9974307583231,9.96759304354012,4.46081218474691));
#37886=CARTESIAN_POINT('Ctrl Pts',(30.9973287715482,9.96899846147698,4.46004957610609));
#37887=CARTESIAN_POINT('Ctrl Pts',(30.9972395295677,9.97020292453311,4.45939628019056));
#37888=CARTESIAN_POINT('Ctrl Pts',(30.997156345061,9.9713256323057,4.45878732801188));
#37889=CARTESIAN_POINT('Ctrl Pts',(30.9970843243445,9.97227315069866,4.45827366363859));
#37890=CARTESIAN_POINT('Ctrl Pts',(30.9970242344315,9.97305438911936,4.45785021755219));
#37891=CARTESIAN_POINT('Ctrl Pts',(30.9969677512095,9.9737887363813,4.4574521873659));
#37892=CARTESIAN_POINT('Ctrl Pts',(30.9969218432233,9.97437583963493,4.45713404448338));
#37893=CARTESIAN_POINT('Ctrl Pts',(30.996883501682,9.9748628795096,4.45687012138836));
#37894=CARTESIAN_POINT('Ctrl Pts',(30.9968451601406,9.97534991938426,4.45660619829334));
#37895=CARTESIAN_POINT('Ctrl Pts',(30.9968144373045,9.97573621414996,4.45639686345456));
#37896=CARTESIAN_POINT('Ctrl Pts',(30.9967839065843,9.97611791660417,4.45619003774767));
#37897=CARTESIAN_POINT('',(30.999709398471,10.0241064018209,4.54380418832777));
#37898=CARTESIAN_POINT('Ctrl Pts',(30.999709398471,10.0241064018209,4.54380418832777));
#37899=CARTESIAN_POINT('Ctrl Pts',(30.9987342345088,10.008110240082,4.51459947146774));
#37900=CARTESIAN_POINT('Ctrl Pts',(30.9977590705465,9.99211407834309,4.4853947546077));
#37901=CARTESIAN_POINT('Ctrl Pts',(30.9967839065843,9.97611791660417,4.45619003774767));
#37902=CARTESIAN_POINT('',(31.,10.,4.55700877125496));
#37903=CARTESIAN_POINT('Ctrl Pts',(30.999709398471,10.0241064018209,4.54380418832777));
#37904=CARTESIAN_POINT('Ctrl Pts',(30.9997130428061,10.0239552686882,4.54388699138558));
#37905=CARTESIAN_POINT('Ctrl Pts',(30.9997167627365,10.023800056336,4.5439720292231));
#37906=CARTESIAN_POINT('Ctrl Pts',(30.9997219491925,10.0235801675738,4.54409250214455));
#37907=CARTESIAN_POINT('Ctrl Pts',(30.9997276919049,10.0233366953556,4.54422589599848));
#37908=CARTESIAN_POINT('Ctrl Pts',(30.999735229715,10.0230141512577,4.54440261195368));
#37909=CARTESIAN_POINT('Ctrl Pts',(30.9997448318797,10.022589181701,4.54463544076275));
#37910=CARTESIAN_POINT('Ctrl Pts',(30.9997558292583,10.0221024632103,4.54490210006752));
#37911=CARTESIAN_POINT('Ctrl Pts',(30.999769492307,10.0214821908588,4.54524192519073));
#37912=CARTESIAN_POINT('Ctrl Pts',(30.9997844949796,10.0207596627717,4.54563775929827));
#37913=CARTESIAN_POINT('Ctrl Pts',(30.9998039339552,10.019823482515,4.54615064188795));
#37914=CARTESIAN_POINT('Ctrl Pts',(30.9998254114386,10.0187197227466,4.54675531137161));
#37915=CARTESIAN_POINT('Ctrl Pts',(30.9998453206045,10.0175879181613,4.54737531334839));
#37916=CARTESIAN_POINT('Ctrl Pts',(30.9998613095551,10.0166789716193,4.54787323380225));
#37917=CARTESIAN_POINT('Ctrl Pts',(30.9998762659289,10.0157556608402,4.54837900388194));
#37918=CARTESIAN_POINT('Ctrl Pts',(30.9998894643458,10.0148680560327,4.54886519675767));
#37919=CARTESIAN_POINT('Ctrl Pts',(30.9999003583534,10.0141354247211,4.54926650161903));
#37920=CARTESIAN_POINT('Ctrl Pts',(30.999910085082,10.0134275501846,4.54965423314624));
#37921=CARTESIAN_POINT('Ctrl Pts',(30.9999188849585,10.0127366990778,4.55003263098948));
#37922=CARTESIAN_POINT('Ctrl Pts',(30.9999281253946,10.0120112609951,4.55042997305517));
#37923=CARTESIAN_POINT('Ctrl Pts',(30.9999364365931,10.0112991469223,4.55082000725131));
#37924=CARTESIAN_POINT('Ctrl Pts',(30.9999442526988,10.0105589532913,4.5512254177633));
#37925=CARTESIAN_POINT('Ctrl Pts',(30.999952520276,10.0097760048231,4.55165424547276));
#37926=CARTESIAN_POINT('Ctrl Pts',(30.9999601897866,10.0089617150539,4.55210023538587));
#37927=CARTESIAN_POINT('Ctrl Pts',(30.9999669593025,10.0081289792326,4.55255632838156));
#37928=CARTESIAN_POINT('Ctrl Pts',(30.999975972948,10.0070201871626,4.55316361857347));
#37929=CARTESIAN_POINT('Ctrl Pts',(30.9999832557419,10.0058807899388,4.55378767133347));
#37930=CARTESIAN_POINT('Ctrl Pts',(30.9999883153679,10.0048341625656,4.55436091900646));
#37931=CARTESIAN_POINT('Ctrl Pts',(30.9999924409198,10.0039807564914,4.55482833755362));
#37932=CARTESIAN_POINT('Ctrl Pts',(30.9999951189592,10.0031932621774,4.55525965958809));
#37933=CARTESIAN_POINT('Ctrl Pts',(30.9999967898708,10.0025338208551,4.55562085125733));
#37934=CARTESIAN_POINT('Ctrl Pts',(30.9999982350687,10.0019634595778,4.55593325167095));
#37935=CARTESIAN_POINT('Ctrl Pts',(30.9999989579243,10.0014899908439,4.55619258717302));
#37936=CARTESIAN_POINT('Ctrl Pts',(30.9999993713266,10.0011213146157,4.55639453011206));
#37937=CARTESIAN_POINT('Ctrl Pts',(30.9999997403671,10.0007922006482,4.55657480276531));
#37938=CARTESIAN_POINT('Ctrl Pts',(30.9999998688457,10.0005469190199,4.55670916222024));
#37939=CARTESIAN_POINT('Ctrl Pts',(30.999999936968,10.0003550550437,4.55681426554227));
#37940=CARTESIAN_POINT('Ctrl Pts',(30.9999999853322,10.0002188389849,4.55688888486672));
#37941=CARTESIAN_POINT('Ctrl Pts',(31.,10.0001088559445,4.55694913671912));
#37942=CARTESIAN_POINT('Ctrl Pts',(31.,10.,4.55700877125496));
#37943=CARTESIAN_POINT('',(31.,9.94795835001335,4.52850438562748));
#37944=CARTESIAN_POINT('Ctrl Pts',(30.7,10.6423370590817,4.2));
#37945=CARTESIAN_POINT('Ctrl Pts',(30.7965969380826,10.5378992444231,4.19999999999999));
#37946=CARTESIAN_POINT('Ctrl Pts',(30.9345468167719,10.3169335076792,4.27686267954766));
#37947=CARTESIAN_POINT('Ctrl Pts',(30.9889170802925,10.0744708831481,4.40289742302579));
#37948=CARTESIAN_POINT('Ctrl Pts',(30.9967839065843,9.97611791660417,4.45619003774767));
#37949=CARTESIAN_POINT('Ctrl Pts',(30.7112855175711,10.6546595286708,4.21735899290232));
#37950=CARTESIAN_POINT('Ctrl Pts',(30.806790559886,10.5514291562489,4.22117275213537));
#37951=CARTESIAN_POINT('Ctrl Pts',(30.9417901498282,10.332363796979,4.30380302692461));
#37952=CARTESIAN_POINT('Ctrl Pts',(30.9917239673576,10.0904674824508,4.4319041792042));
#37953=CARTESIAN_POINT('Ctrl Pts',(30.9977590705465,9.99211407834309,4.4853947546077));
#37954=CARTESIAN_POINT('Ctrl Pts',(30.7225710351422,10.66698199826,4.23471798580464));
#37955=CARTESIAN_POINT('Ctrl Pts',(30.8169841816893,10.5649590680747,4.24234550427075));
#37956=CARTESIAN_POINT('Ctrl Pts',(30.9490334828845,10.3477940862788,4.33074337430155));
#37957=CARTESIAN_POINT('Ctrl Pts',(30.9945308544227,10.1064640817536,4.46091093538261));
#37958=CARTESIAN_POINT('Ctrl Pts',(30.9987342345088,10.008110240082,4.51459947146774));
#37959=CARTESIAN_POINT('Ctrl Pts',(30.7338565527132,10.6793044678492,4.25207697870696));
#37960=CARTESIAN_POINT('Ctrl Pts',(30.8271778034927,10.5784889799005,4.26351825640613));
#37961=CARTESIAN_POINT('Ctrl Pts',(30.9562768159408,10.3632243755785,4.3576837216785));
#37962=CARTESIAN_POINT('Ctrl Pts',(30.9973377414878,10.1224606810563,4.48991769156102));
#37963=CARTESIAN_POINT('Ctrl Pts',(30.999709398471,10.0241064018209,4.54380418832777));
#37964=CARTESIAN_POINT('Ctrl Pts',(30.9967839065843,9.97611791660417,4.45619003774767));
#37965=CARTESIAN_POINT('Ctrl Pts',(30.9889170802925,10.0744708831481,4.40289742302579));
#37966=CARTESIAN_POINT('Ctrl Pts',(30.9345468167719,10.3169335076792,4.27686267954766));
#37967=CARTESIAN_POINT('Ctrl Pts',(30.7965969380826,10.5378992444231,4.19999999999999));
#37968=CARTESIAN_POINT('Ctrl Pts',(30.7,10.6423370590817,4.2));
#37969=CARTESIAN_POINT('',(30.7338565527132,10.6793044678492,4.25207697870696));
#37970=CARTESIAN_POINT('',(30.7,10.6423370590817,4.2));
#37971=CARTESIAN_POINT('Ctrl Pts',(30.7338565527132,10.6793044678492,4.25207697870696));
#37972=CARTESIAN_POINT('Ctrl Pts',(30.8271778034927,10.5784889799005,4.26351825640613));
#37973=CARTESIAN_POINT('Ctrl Pts',(30.9562768159408,10.3632243755785,4.3576837216785));
#37974=CARTESIAN_POINT('Ctrl Pts',(30.9973377414878,10.1224606810563,4.48991769156102));
#37975=CARTESIAN_POINT('Ctrl Pts',(30.999709398471,10.0241064018209,4.54380418832777));
#37976=CARTESIAN_POINT('Origin',(15.,-10.975,4.225));
#37977=CARTESIAN_POINT('',(30.,-11.,4.25));
#37978=CARTESIAN_POINT('',(30.,-10.95,4.2));
#37979=CARTESIAN_POINT('',(21.05,-11.,4.25));
#37980=CARTESIAN_POINT('',(15.,-11.,4.25));
#37981=CARTESIAN_POINT('',(21.05,-11.,4.25));
#37982=CARTESIAN_POINT('Origin',(21.025,-10.975,4.2));
#37983=CARTESIAN_POINT('',(21.05,-11.,4.85));
#37984=CARTESIAN_POINT('',(21.05,-11.,4.2));
#37985=CARTESIAN_POINT('',(21.,-10.95,4.8));
#37986=CARTESIAN_POINT('',(21.05,-11.,4.85));
#37987=CARTESIAN_POINT('',(21.,-10.95,4.2));
#37988=CARTESIAN_POINT('Origin',(18.95,-11.,4.25));
#37989=CARTESIAN_POINT('',(19.,-10.95,4.25));
#37990=CARTESIAN_POINT('',(18.95,-10.95,4.2));
#37991=CARTESIAN_POINT('',(19.,-10.95,4.25));
#37992=CARTESIAN_POINT('',(18.95,-11.,4.25));
#37993=CARTESIAN_POINT('',(18.95,-11.,4.25));
#37994=CARTESIAN_POINT('',(18.95,-10.95,4.2));
#37995=CARTESIAN_POINT('Origin',(18.975,-10.975,4.2));
#37996=CARTESIAN_POINT('',(18.95,-11.,4.85));
#37997=CARTESIAN_POINT('',(18.95,-11.,4.2));
#37998=CARTESIAN_POINT('',(19.,-10.95,4.8));
#37999=CARTESIAN_POINT('',(19.,-10.95,4.2));
#38000=CARTESIAN_POINT('',(19.,-10.95,4.8));
#38001=CARTESIAN_POINT('Origin',(18.95,11.,4.25));
#38002=CARTESIAN_POINT('',(18.95,10.95,4.2));
#38003=CARTESIAN_POINT('',(19.,10.95,4.25));
#38004=CARTESIAN_POINT('',(18.95,10.95,4.2));
#38005=CARTESIAN_POINT('',(18.95,11.,4.25));
#38006=CARTESIAN_POINT('',(18.95,11.,4.25));
#38007=CARTESIAN_POINT('',(19.,10.95,4.25));
#38008=CARTESIAN_POINT('Origin',(25.,10.975,4.225));
#38009=CARTESIAN_POINT('',(10.,10.95,4.2));
#38010=CARTESIAN_POINT('',(10.,11.,4.25));
#38011=CARTESIAN_POINT('',(10.,10.95,4.2));
#38012=CARTESIAN_POINT('',(25.,11.,4.25));
#38013=CARTESIAN_POINT('',(25.,10.95,4.2));
#38014=CARTESIAN_POINT('Origin',(10.,10.,4.225));
#38015=CARTESIAN_POINT('',(9.05,10.,4.2));
#38016=CARTESIAN_POINT('',(9.,10.,4.25));
#38017=CARTESIAN_POINT('',(9.05,10.,4.2));
#38018=CARTESIAN_POINT('Origin',(10.,10.,4.25));
#38019=CARTESIAN_POINT('Origin',(10.,10.,4.2));
#38020=CARTESIAN_POINT('Origin',(9.025,5.,4.225));
#38021=CARTESIAN_POINT('',(9.05,-10.,4.2));
#38022=CARTESIAN_POINT('',(9.,-10.,4.25));
#38023=CARTESIAN_POINT('',(9.05,-10.,4.2));
#38024=CARTESIAN_POINT('',(9.,5.,4.25));
#38025=CARTESIAN_POINT('',(9.05,5.,4.2));
#38026=CARTESIAN_POINT('Origin',(10.,-10.,4.225));
#38027=CARTESIAN_POINT('',(10.,-10.95,4.2));
#38028=CARTESIAN_POINT('',(10.,-11.,4.25));
#38029=CARTESIAN_POINT('',(10.,-10.95,4.2));
#38030=CARTESIAN_POINT('Origin',(10.,-10.,4.25));
#38031=CARTESIAN_POINT('Origin',(10.,-10.,4.2));
#38032=CARTESIAN_POINT('Origin',(15.,-10.975,4.225));
#38033=CARTESIAN_POINT('',(15.,-10.95,4.2));
#38034=CARTESIAN_POINT('',(15.,-11.,4.25));
#38035=CARTESIAN_POINT('Origin',(18.975,10.975,4.2));
#38036=CARTESIAN_POINT('',(19.,10.95,4.8));
#38037=CARTESIAN_POINT('',(19.,10.95,4.2));
#38038=CARTESIAN_POINT('',(18.95,11.,4.85));
#38039=CARTESIAN_POINT('',(18.95,11.,4.2));
#38040=CARTESIAN_POINT('',(18.95,11.,4.85));
#38041=CARTESIAN_POINT('Origin',(18.975,5.55,4.225));
#38042=CARTESIAN_POINT('',(18.95,5.55,4.2));
#38043=CARTESIAN_POINT('',(19.,5.55,4.25));
#38044=CARTESIAN_POINT('Origin',(25.,10.975,4.825));
#38045=CARTESIAN_POINT('',(25.,10.95,4.8));
#38046=CARTESIAN_POINT('',(25.,11.,4.85));
#38047=CARTESIAN_POINT('Origin',(15.,-10.975,4.825));
#38048=CARTESIAN_POINT('',(15.,-11.,4.85));
#38049=CARTESIAN_POINT('',(15.,-10.95,4.8));
#38050=CARTESIAN_POINT('Origin',(30.,10.,4.225));
#38051=CARTESIAN_POINT('',(30.7,10.7141428428543,4.25));
#38052=CARTESIAN_POINT('Origin',(30.,10.,4.25));
#38053=CARTESIAN_POINT('',(30.7,10.7141428428543,4.25));
#38054=CARTESIAN_POINT('Origin',(30.,-10.,4.225));
#38055=CARTESIAN_POINT('',(30.7,-10.7141428428543,4.25));
#38056=CARTESIAN_POINT('',(30.665,-10.6784357007116,4.2));
#38057=CARTESIAN_POINT('Origin',(30.,-10.,4.25));
#38058=CARTESIAN_POINT('Ctrl Pts',(30.7338565527132,10.6793044678492,4.25207697870696));
#38059=CARTESIAN_POINT('Ctrl Pts',(30.7228338070625,10.6912124038448,4.25072557918173));
#38060=CARTESIAN_POINT('Ctrl Pts',(30.7115415847052,10.7028298270137,4.25));
#38061=CARTESIAN_POINT('Ctrl Pts',(30.7,10.7141428428543,4.25));
#38062=CARTESIAN_POINT('Ctrl Pts',(30.7225710351422,10.66698199826,4.23471798580464));
#38063=CARTESIAN_POINT('Ctrl Pts',(30.7114193189812,10.6790325526684,4.23381705278782));
#38064=CARTESIAN_POINT('Ctrl Pts',(30.7000220784993,10.6907832001958,4.23333333333333));
#38065=CARTESIAN_POINT('Ctrl Pts',(30.6883333333333,10.70224046214,4.23333333333333));
#38066=CARTESIAN_POINT('Ctrl Pts',(30.7112855175711,10.6546595286708,4.21735899290232));
#38067=CARTESIAN_POINT('Ctrl Pts',(30.7000048309,10.666852701492,4.21690852639391));
#38068=CARTESIAN_POINT('Ctrl Pts',(30.6885025722933,10.678736573378,4.21666666666667));
#38069=CARTESIAN_POINT('Ctrl Pts',(30.6766666666667,10.6903380814258,4.21666666666667));
#38070=CARTESIAN_POINT('Ctrl Pts',(30.7,10.6423370590817,4.2));
#38071=CARTESIAN_POINT('Ctrl Pts',(30.6885903428187,10.6546728503156,4.2));
#38072=CARTESIAN_POINT('Ctrl Pts',(30.6769830660874,10.6666899465601,4.2));
#38073=CARTESIAN_POINT('Ctrl Pts',(30.665,10.6784357007116,4.2));
#38074=CARTESIAN_POINT('Ctrl Pts',(30.7,10.7141428428543,4.25));
#38075=CARTESIAN_POINT('Ctrl Pts',(30.7115415847052,10.7028298270137,4.25));
#38076=CARTESIAN_POINT('Ctrl Pts',(30.7228338070625,10.6912124038448,4.25072557918173));
#38077=CARTESIAN_POINT('Ctrl Pts',(30.7338565527132,10.6793044678492,4.25207697870696));
#38078=CARTESIAN_POINT('Ctrl Pts',(30.9967838963896,-9.97611804405966,4.45618996868547));
#38079=CARTESIAN_POINT('Ctrl Pts',(30.9889170789375,-10.0744707456924,4.40289749968711));
#38080=CARTESIAN_POINT('Ctrl Pts',(30.9345467803032,-10.3169335644504,4.27686265785453));
#38081=CARTESIAN_POINT('Ctrl Pts',(30.7965969202196,-10.5378992637361,4.19999999999999));
#38082=CARTESIAN_POINT('Ctrl Pts',(30.7,-10.6423370590817,4.2));
#38083=CARTESIAN_POINT('Ctrl Pts',(30.9977590627279,-9.99211420570491,4.4853946853406));
#38084=CARTESIAN_POINT('Ctrl Pts',(30.9917239593499,-10.0904675123771,4.4319041637732));
#38085=CARTESIAN_POINT('Ctrl Pts',(30.9417901139861,-10.3323638606833,4.30380299959424));
#38086=CARTESIAN_POINT('Ctrl Pts',(30.8067905422249,-10.5514291753386,4.22117275143012));
#38087=CARTESIAN_POINT('Ctrl Pts',(30.7112855175711,-10.6546595286708,4.21735899290232));
#38088=CARTESIAN_POINT('Ctrl Pts',(30.9987342290661,-10.0081103673502,4.51459940199573));
#38089=CARTESIAN_POINT('Ctrl Pts',(30.9945308397623,-10.1064642790619,4.46091082785928));
#38090=CARTESIAN_POINT('Ctrl Pts',(30.9490334476689,-10.3477941569161,4.33074334133394));
#38091=CARTESIAN_POINT('Ctrl Pts',(30.8169841642302,-10.5649590869411,4.24234550286025));
#38092=CARTESIAN_POINT('Ctrl Pts',(30.7225710351422,-10.66698199826,4.23471798580464));
#38093=CARTESIAN_POINT('Ctrl Pts',(30.9997093954044,-10.0241065289954,4.54380411865086));
#38094=CARTESIAN_POINT('Ctrl Pts',(30.9973377201748,-10.1224610457467,4.48991749194537));
#38095=CARTESIAN_POINT('Ctrl Pts',(30.9562767813518,-10.363224453149,4.35768368307365));
#38096=CARTESIAN_POINT('Ctrl Pts',(30.8271777862355,-10.5784889985436,4.26351825429037));
#38097=CARTESIAN_POINT('Ctrl Pts',(30.7338565527132,-10.6793044678492,4.25207697870696));
#38098=CARTESIAN_POINT('',(30.7338565527132,-10.6793044678492,4.25207697870696));
#38099=CARTESIAN_POINT('Ctrl Pts',(30.9997093954044,-10.0241065289954,4.54380411865086));
#38100=CARTESIAN_POINT('Ctrl Pts',(30.9973377201748,-10.1224610457467,4.48991749194537));
#38101=CARTESIAN_POINT('Ctrl Pts',(30.9562767813518,-10.363224453149,4.35768368307365));
#38102=CARTESIAN_POINT('Ctrl Pts',(30.8271777862355,-10.5784889985436,4.26351825429037));
#38103=CARTESIAN_POINT('Ctrl Pts',(30.7338565527132,-10.6793044678492,4.25207697870696));
#38104=CARTESIAN_POINT('',(30.7338565527132,-10.6793044678492,4.25207697870696));
#38105=CARTESIAN_POINT('Ctrl Pts',(30.7,-10.6423370590817,4.2));
#38106=CARTESIAN_POINT('Ctrl Pts',(30.7965969202196,-10.5378992637361,4.19999999999999));
#38107=CARTESIAN_POINT('Ctrl Pts',(30.9345467803032,-10.3169335644504,4.27686265785453));
#38108=CARTESIAN_POINT('Ctrl Pts',(30.9889170789375,-10.0744707456924,4.40289749968711));
#38109=CARTESIAN_POINT('Ctrl Pts',(30.9967838963896,-9.97611804405966,4.45618996868547));
#38110=CARTESIAN_POINT('Ctrl Pts',(30.7,-10.7141428428543,4.25));
#38111=CARTESIAN_POINT('Ctrl Pts',(30.7115415847052,-10.7028298270137,4.25));
#38112=CARTESIAN_POINT('Ctrl Pts',(30.7228338070625,-10.6912124038448,4.25072557918172));
#38113=CARTESIAN_POINT('Ctrl Pts',(30.7338565527132,-10.6793044678492,4.25207697870696));
#38114=CARTESIAN_POINT('Ctrl Pts',(30.6883333333333,-10.70224046214,4.23333333333333));
#38115=CARTESIAN_POINT('Ctrl Pts',(30.7000220784993,-10.6907832001958,4.23333333333333));
#38116=CARTESIAN_POINT('Ctrl Pts',(30.7114193189812,-10.6790325526684,4.23381705278782));
#38117=CARTESIAN_POINT('Ctrl Pts',(30.7225710351422,-10.66698199826,4.23471798580464));
#38118=CARTESIAN_POINT('Ctrl Pts',(30.6766666666667,-10.6903380814258,4.21666666666667));
#38119=CARTESIAN_POINT('Ctrl Pts',(30.6885025722933,-10.678736573378,4.21666666666667));
#38120=CARTESIAN_POINT('Ctrl Pts',(30.7000048309,-10.666852701492,4.21690852639391));
#38121=CARTESIAN_POINT('Ctrl Pts',(30.7112855175711,-10.6546595286708,4.21735899290232));
#38122=CARTESIAN_POINT('Ctrl Pts',(30.665,-10.6784357007116,4.2));
#38123=CARTESIAN_POINT('Ctrl Pts',(30.6769830660874,-10.6666899465601,4.2));
#38124=CARTESIAN_POINT('Ctrl Pts',(30.6885903428187,-10.6546728503156,4.2));
#38125=CARTESIAN_POINT('Ctrl Pts',(30.7,-10.6423370590817,4.2));
#38126=CARTESIAN_POINT('Ctrl Pts',(30.7338565527132,-10.6793044678492,4.25207697870696));
#38127=CARTESIAN_POINT('Ctrl Pts',(30.7228338070625,-10.6912124038448,4.25072557918172));
#38128=CARTESIAN_POINT('Ctrl Pts',(30.7115415847052,-10.7028298270137,4.25));
#38129=CARTESIAN_POINT('Ctrl Pts',(30.7,-10.7141428428543,4.25));
#38130=CARTESIAN_POINT('Origin',(10.,-11.,4.2));
#38131=CARTESIAN_POINT('',(30.,-11.,6.15));
#38132=CARTESIAN_POINT('',(30.,-11.,4.2));
#38133=CARTESIAN_POINT('',(10.,-11.,6.15));
#38134=CARTESIAN_POINT('',(15.,-11.,6.15));
#38135=CARTESIAN_POINT('',(10.,-11.,4.2));
#38136=CARTESIAN_POINT('Origin',(30.,-10.,4.2));
#38137=CARTESIAN_POINT('',(31.,-10.,5.84299122874504));
#38138=CARTESIAN_POINT('',(31.,-10.,4.2));
#38139=CARTESIAN_POINT('',(30.9997094022748,-10.0241062440753,5.85619572522048));
#38140=CARTESIAN_POINT('Ctrl Pts',(30.9997094022748,-10.0241062440753,5.85619572522048));
#38141=CARTESIAN_POINT('Ctrl Pts',(30.9997130467291,-10.0239551050077,5.85611291886692));
#38142=CARTESIAN_POINT('Ctrl Pts',(30.9997167667759,-10.0237998867075,5.8560278777443));
#38143=CARTESIAN_POINT('Ctrl Pts',(30.9997219533132,-10.023579992868,5.85590740213001));
#38144=CARTESIAN_POINT('Ctrl Pts',(30.9997276961238,-10.0233365146857,5.8557740051069));
#38145=CARTESIAN_POINT('Ctrl Pts',(30.9997352339929,-10.0230139654796,5.85559728658946));
#38146=CARTESIAN_POINT('Ctrl Pts',(30.9997448361474,-10.0225889928205,5.85536445634685));
#38147=CARTESIAN_POINT('Ctrl Pts',(30.9997558335613,-10.0221022686959,5.85509779426031));
#38148=CARTESIAN_POINT('Ctrl Pts',(30.9997694965754,-10.0214819922295,5.85475796721774));
#38149=CARTESIAN_POINT('Ctrl Pts',(30.9997844991176,-10.020759463484,5.85436213274578));
#38150=CARTESIAN_POINT('Ctrl Pts',(30.9998039371891,-10.0198233177775,5.85384926907949));
#38151=CARTESIAN_POINT('Ctrl Pts',(30.9998254134561,-10.0187196114834,5.8532446282723));
#38152=CARTESIAN_POINT('Ctrl Pts',(30.9998453215427,-10.017587864828,5.85262465607974));
#38153=CARTESIAN_POINT('Ctrl Pts',(30.9998613100668,-10.0166789397704,5.85212674582915));
#38154=CARTESIAN_POINT('Ctrl Pts',(30.9998762660452,-10.0157556522058,5.85162098603055));
#38155=CARTESIAN_POINT('Ctrl Pts',(30.9998894641422,-10.0148680697274,5.85113480211444));
#38156=CARTESIAN_POINT('Ctrl Pts',(30.9999003578812,-10.014135457153,5.85073350481631));
#38157=CARTESIAN_POINT('Ctrl Pts',(30.9999100843927,-10.0134276007098,5.85034577993147));
#38158=CARTESIAN_POINT('Ctrl Pts',(30.999918884115,-10.0127367653004,5.84996738720872));
#38159=CARTESIAN_POINT('Ctrl Pts',(30.9999281242885,-10.0120113516037,5.84957005484841));
#38160=CARTESIAN_POINT('Ctrl Pts',(30.9999364353128,-10.0112992590878,5.84918002861482));
#38161=CARTESIAN_POINT('Ctrl Pts',(30.9999442513311,-10.0105590828167,5.84877462429034));
#38162=CARTESIAN_POINT('Ctrl Pts',(30.9999525187802,-10.0097761560831,5.84834580497266));
#38163=CARTESIAN_POINT('Ctrl Pts',(30.9999601882674,-10.0089618835122,5.84789982155921));
#38164=CARTESIAN_POINT('Ctrl Pts',(30.9999669578405,-10.0081291590671,5.84744373291581));
#38165=CARTESIAN_POINT('Ctrl Pts',(30.9999759712677,-10.0070204183844,5.84683646836768));
#38166=CARTESIAN_POINT('Ctrl Pts',(30.9999832541069,-10.0058810641504,5.84621243851916));
#38167=CARTESIAN_POINT('Ctrl Pts',(30.999988313939,-10.0048344581344,5.84563920390379));
#38168=CARTESIAN_POINT('Ctrl Pts',(30.9999924398875,-10.003981022191,5.84517177010603));
#38169=CARTESIAN_POINT('Ctrl Pts',(30.999995118254,-10.0031934906294,5.84474043007898));
#38170=CARTESIAN_POINT('Ctrl Pts',(30.9999967893852,-10.0025340125065,5.84437922167547));
#38171=CARTESIAN_POINT('Ctrl Pts',(30.9999982347598,-10.0019636246513,5.84406680966457));
#38172=CARTESIAN_POINT('Ctrl Pts',(30.9999989577288,-10.0014901279877,5.84380746257457));
#38173=CARTESIAN_POINT('Ctrl Pts',(30.9999993711998,-10.001121427621,5.84360551058622));
#38174=CARTESIAN_POINT('Ctrl Pts',(30.9999997402998,-10.0007922938583,5.84342523081487));
#38175=CARTESIAN_POINT('Ctrl Pts',(30.9999998688065,-10.0005469945696,5.84329086577593));
#38176=CARTESIAN_POINT('Ctrl Pts',(30.9999999369451,-10.0003551195025,5.84318576061118));
#38177=CARTESIAN_POINT('Ctrl Pts',(30.9999999853286,-10.000218873612,5.84311112795059));
#38178=CARTESIAN_POINT('Ctrl Pts',(31.,-10.0001088728919,5.84305086948946));
#38179=CARTESIAN_POINT('Ctrl Pts',(31.,-10.,5.84299122874504));
#38180=CARTESIAN_POINT('',(30.7338565527125,-10.6793044678499,6.14792302129313));
#38181=CARTESIAN_POINT('Ctrl Pts',(30.7338565527125,-10.6793044678499,6.14792302129313));
#38182=CARTESIAN_POINT('Ctrl Pts',(30.7622591025997,-10.6486210286339,6.14444084056899));
#38183=CARTESIAN_POINT('Ctrl Pts',(30.7899347430608,-10.6147354943559,6.13657883580837));
#38184=CARTESIAN_POINT('Ctrl Pts',(30.8465633390414,-10.5350521462962,6.11173493670335));
#38185=CARTESIAN_POINT('Ctrl Pts',(30.8872065032282,-10.4658719010602,6.08407025994295));
#38186=CARTESIAN_POINT('Ctrl Pts',(30.9368867620569,-10.3553346508213,6.03274417903868));
#38187=CARTESIAN_POINT('Ctrl Pts',(30.9615371967044,-10.2795901391215,5.99406746301422));
#38188=CARTESIAN_POINT('Ctrl Pts',(30.989705810262,-10.1599951404466,5.93078512444313));
#38189=CARTESIAN_POINT('Ctrl Pts',(30.9981384709031,-10.0892542969071,5.89188916163067));
#38190=CARTESIAN_POINT('Ctrl Pts',(30.9997094022748,-10.0241062440753,5.85619572522048));
#38191=CARTESIAN_POINT('',(30.7,-10.7141428428543,6.15));
#38192=CARTESIAN_POINT('Ctrl Pts',(30.7,-10.7141428428543,6.15));
#38193=CARTESIAN_POINT('Ctrl Pts',(30.7112905851662,-10.7030758557726,6.15));
#38194=CARTESIAN_POINT('Ctrl Pts',(30.7226212987117,-10.6914419778475,6.14930047455236));
#38195=CARTESIAN_POINT('Ctrl Pts',(30.7338565527125,-10.6793044678499,6.14792302129313));
#38196=CARTESIAN_POINT('Origin',(30.,-10.,6.15));
#38197=CARTESIAN_POINT('Origin',(31.,0.,14.5));
#38198=CARTESIAN_POINT('',(31.,0.,4.5));
#38199=CARTESIAN_POINT('',(31.,10.,5.84299122874504));
#38200=CARTESIAN_POINT('',(31.,10.,4.2));
#38201=CARTESIAN_POINT('',(31.,9.89591670002669,5.9));
#38202=CARTESIAN_POINT('',(31.,9.94795835001334,5.87149561437252));
#38203=CARTESIAN_POINT('',(31.,7.76915840380663,5.9));
#38204=CARTESIAN_POINT('',(31.,0.,5.9));
#38205=CARTESIAN_POINT('',(31.,3.52895676585423,21.8971243613659));
#38206=CARTESIAN_POINT('',(31.,6.41964359742627,10.9913513149805));
#38207=CARTESIAN_POINT('',(31.,-3.52895676585423,21.8971243613659));
#38208=CARTESIAN_POINT('Origin',(31.,0.,26.5));
#38209=CARTESIAN_POINT('',(31.,-7.76915840380663,5.9));
#38210=CARTESIAN_POINT('',(31.,-4.21964359742627,19.2913513149805));
#38211=CARTESIAN_POINT('',(31.,-9.89591670002669,5.9));
#38212=CARTESIAN_POINT('',(31.,0.,5.9));
#38213=CARTESIAN_POINT('',(31.,-9.94795835001334,5.87149561437252));
#38214=CARTESIAN_POINT('',(31.,-4.8,14.));
#38215=CARTESIAN_POINT('',(31.,-4.8,5.9));
#38216=CARTESIAN_POINT('',(31.,-4.8,10.35));
#38217=CARTESIAN_POINT('',(31.,4.8,14.));
#38218=CARTESIAN_POINT('Origin',(31.,0.,14.));
#38219=CARTESIAN_POINT('',(31.,4.8,5.9));
#38220=CARTESIAN_POINT('',(31.,4.8,14.25));
#38221=CARTESIAN_POINT('',(31.,0.,5.9));
#38222=CARTESIAN_POINT('Origin',(30.7,0.,4.5));
#38223=CARTESIAN_POINT('Origin',(19.,11.1,4.2));
#38224=CARTESIAN_POINT('',(19.,11.1,4.8));
#38225=CARTESIAN_POINT('Origin',(21.,-11.1,4.2));
#38226=CARTESIAN_POINT('',(21.,-11.1,4.8));
#38227=CARTESIAN_POINT('Origin',(20.,0.,4.8));
#38228=CARTESIAN_POINT('Origin',(20.,0.,4.2));
#38229=CARTESIAN_POINT('',(10.4,9.,4.2));
#38230=CARTESIAN_POINT('',(10.4,9.4,4.2));
#38231=CARTESIAN_POINT('',(10.4,4.5,4.2));
#38232=CARTESIAN_POINT('',(11.6,9.,4.2));
#38233=CARTESIAN_POINT('Origin',(11.,9.,4.2));
#38234=CARTESIAN_POINT('',(11.6,9.4,4.2));
#38235=CARTESIAN_POINT('',(11.6,4.7,4.2));
#38236=CARTESIAN_POINT('Origin',(11.,9.4,4.2));
#38237=CARTESIAN_POINT('',(10.4,-9.4,4.2));
#38238=CARTESIAN_POINT('',(10.4,-9.,4.2));
#38239=CARTESIAN_POINT('',(10.4,-4.7,4.2));
#38240=CARTESIAN_POINT('',(11.6,-9.4,4.2));
#38241=CARTESIAN_POINT('Origin',(11.,-9.4,4.2));
#38242=CARTESIAN_POINT('',(11.6,-9.,4.2));
#38243=CARTESIAN_POINT('',(11.6,-4.5,4.2));
#38244=CARTESIAN_POINT('Origin',(11.,-9.,4.2));
#38245=CARTESIAN_POINT('Origin',(28.425,-4.7,4.225));
#38246=CARTESIAN_POINT('',(28.45,-9.4,4.25));
#38247=CARTESIAN_POINT('',(28.45,-9.4,4.25));
#38248=CARTESIAN_POINT('',(28.45,-9.,4.25));
#38249=CARTESIAN_POINT('',(28.4,-9.,4.2));
#38250=CARTESIAN_POINT('',(28.45,-4.7,4.25));
#38251=CARTESIAN_POINT('Origin',(29.,-9.4,4.225));
#38252=CARTESIAN_POINT('',(29.55,-9.4,4.25));
#38253=CARTESIAN_POINT('',(29.55,-9.4,4.25));
#38254=CARTESIAN_POINT('Origin',(29.,-9.4,4.25));
#38255=CARTESIAN_POINT('Origin',(29.575,-4.5,4.225));
#38256=CARTESIAN_POINT('',(29.55,-9.,4.25));
#38257=CARTESIAN_POINT('',(29.55,-9.,4.25));
#38258=CARTESIAN_POINT('',(29.55,-4.5,4.25));
#38259=CARTESIAN_POINT('Origin',(29.,-9.,4.225));
#38260=CARTESIAN_POINT('Origin',(29.,-9.,4.25));
#38261=CARTESIAN_POINT('Origin',(29.,-9.4,6.2));
#38262=CARTESIAN_POINT('',(28.45,-9.4,6.15));
#38263=CARTESIAN_POINT('',(28.45,-9.4,6.2));
#38264=CARTESIAN_POINT('',(29.55,-9.4,6.15));
#38265=CARTESIAN_POINT('Origin',(29.,-9.4,6.15));
#38266=CARTESIAN_POINT('',(29.55,-9.4,6.2));
#38267=CARTESIAN_POINT('Origin',(28.45,-9.4,6.2));
#38268=CARTESIAN_POINT('',(28.45,-9.,6.15));
#38269=CARTESIAN_POINT('',(28.45,-9.,6.2));
#38270=CARTESIAN_POINT('',(28.45,-4.7,6.15));
#38271=CARTESIAN_POINT('Origin',(10.425,4.5,4.225));
#38272=CARTESIAN_POINT('',(10.45,9.,4.25));
#38273=CARTESIAN_POINT('',(10.45,9.,4.25));
#38274=CARTESIAN_POINT('',(10.45,9.4,4.25));
#38275=CARTESIAN_POINT('',(10.4,9.4,4.2));
#38276=CARTESIAN_POINT('',(10.45,4.5,4.25));
#38277=CARTESIAN_POINT('Origin',(11.,9.,4.225));
#38278=CARTESIAN_POINT('',(11.55,9.,4.25));
#38279=CARTESIAN_POINT('',(11.55,9.,4.25));
#38280=CARTESIAN_POINT('Origin',(11.,9.,4.25));
#38281=CARTESIAN_POINT('Origin',(11.575,4.7,4.225));
#38282=CARTESIAN_POINT('',(11.55,9.4,4.25));
#38283=CARTESIAN_POINT('',(11.55,9.4,4.25));
#38284=CARTESIAN_POINT('',(11.55,4.7,4.25));
#38285=CARTESIAN_POINT('Origin',(11.,9.4,4.225));
#38286=CARTESIAN_POINT('Origin',(11.,9.4,4.25));
#38287=CARTESIAN_POINT('Origin',(11.,9.,6.2));
#38288=CARTESIAN_POINT('',(10.45,9.,6.15));
#38289=CARTESIAN_POINT('',(10.45,9.,6.2));
#38290=CARTESIAN_POINT('',(11.55,9.,6.15));
#38291=CARTESIAN_POINT('Origin',(11.,9.,6.15));
#38292=CARTESIAN_POINT('',(11.55,9.,6.2));
#38293=CARTESIAN_POINT('Origin',(10.45,9.,6.2));
#38294=CARTESIAN_POINT('',(10.45,9.4,6.15));
#38295=CARTESIAN_POINT('',(10.45,9.4,6.2));
#38296=CARTESIAN_POINT('',(10.45,4.5,6.15));
#38297=CARTESIAN_POINT('Origin',(10.425,-4.7,4.225));
#38298=CARTESIAN_POINT('',(10.45,-9.4,4.25));
#38299=CARTESIAN_POINT('',(10.45,-9.4,4.25));
#38300=CARTESIAN_POINT('',(10.45,-9.,4.25));
#38301=CARTESIAN_POINT('',(10.4,-9.,4.2));
#38302=CARTESIAN_POINT('',(10.45,-4.7,4.25));
#38303=CARTESIAN_POINT('Origin',(11.,-9.4,4.225));
#38304=CARTESIAN_POINT('',(11.55,-9.4,4.25));
#38305=CARTESIAN_POINT('',(11.55,-9.4,4.25));
#38306=CARTESIAN_POINT('Origin',(11.,-9.4,4.25));
#38307=CARTESIAN_POINT('Origin',(11.575,-4.5,4.225));
#38308=CARTESIAN_POINT('',(11.55,-9.,4.25));
#38309=CARTESIAN_POINT('',(11.55,-9.,4.25));
#38310=CARTESIAN_POINT('',(11.55,-4.5,4.25));
#38311=CARTESIAN_POINT('Origin',(11.,-9.,4.225));
#38312=CARTESIAN_POINT('Origin',(11.,-9.,4.25));
#38313=CARTESIAN_POINT('Origin',(11.,-9.4,6.2));
#38314=CARTESIAN_POINT('',(10.45,-9.4,6.15));
#38315=CARTESIAN_POINT('',(10.45,-9.4,6.2));
#38316=CARTESIAN_POINT('',(11.55,-9.4,6.15));
#38317=CARTESIAN_POINT('Origin',(11.,-9.4,6.15));
#38318=CARTESIAN_POINT('',(11.55,-9.4,6.2));
#38319=CARTESIAN_POINT('Origin',(10.45,-9.4,6.2));
#38320=CARTESIAN_POINT('',(10.45,-9.,6.15));
#38321=CARTESIAN_POINT('',(10.45,-9.,6.2));
#38322=CARTESIAN_POINT('',(10.45,-4.7,6.15));
#38323=CARTESIAN_POINT('Origin',(28.425,4.5,4.225));
#38324=CARTESIAN_POINT('',(28.45,9.,4.25));
#38325=CARTESIAN_POINT('',(28.45,9.,4.25));
#38326=CARTESIAN_POINT('',(28.45,9.4,4.25));
#38327=CARTESIAN_POINT('',(28.4,9.4,4.2));
#38328=CARTESIAN_POINT('',(28.45,4.5,4.25));
#38329=CARTESIAN_POINT('Origin',(29.,9.,4.225));
#38330=CARTESIAN_POINT('',(29.55,9.,4.25));
#38331=CARTESIAN_POINT('',(29.55,9.,4.25));
#38332=CARTESIAN_POINT('Origin',(29.,9.,4.25));
#38333=CARTESIAN_POINT('Origin',(29.575,4.7,4.225));
#38334=CARTESIAN_POINT('',(29.55,9.4,4.25));
#38335=CARTESIAN_POINT('',(29.55,9.4,4.25));
#38336=CARTESIAN_POINT('',(29.55,4.7,4.25));
#38337=CARTESIAN_POINT('Origin',(29.,9.4,4.225));
#38338=CARTESIAN_POINT('Origin',(29.,9.4,4.25));
#38339=CARTESIAN_POINT('Origin',(29.,9.,6.2));
#38340=CARTESIAN_POINT('',(28.45,9.,6.15));
#38341=CARTESIAN_POINT('',(28.45,9.,6.2));
#38342=CARTESIAN_POINT('',(29.55,9.,6.15));
#38343=CARTESIAN_POINT('Origin',(29.,9.,6.15));
#38344=CARTESIAN_POINT('',(29.55,9.,6.2));
#38345=CARTESIAN_POINT('Origin',(28.45,9.,6.2));
#38346=CARTESIAN_POINT('',(28.45,9.4,6.15));
#38347=CARTESIAN_POINT('',(28.45,9.4,6.2));
#38348=CARTESIAN_POINT('',(28.45,4.5,6.15));
#38349=CARTESIAN_POINT('Origin',(8.025,-3.53553390593274,30.0355339059327));
#38350=CARTESIAN_POINT('',(8.,-3.53553390593274,30.3905339059327));
#38351=CARTESIAN_POINT('Origin',(8.,-3.53553390593274,30.0355339059327));
#38352=CARTESIAN_POINT('',(8.05,-3.53553390593274,30.3405339059327));
#38353=CARTESIAN_POINT('',(8.025,-3.53553390593274,30.3655339059327));
#38354=CARTESIAN_POINT('',(8.05,-3.53553390593274,29.7305339059327));
#38355=CARTESIAN_POINT('Origin',(8.05,-3.53553390593274,30.0355339059327));
#38356=CARTESIAN_POINT('Origin',(8.05,-3.53553390593274,30.0355339059327));
#38357=CARTESIAN_POINT('Origin',(8.,-3.53553390593274,30.0355339059327));
#38358=CARTESIAN_POINT('Origin',(8.685,-3.53553390593274,30.0355339059327));
#38359=CARTESIAN_POINT('',(9.4,-3.53553390593274,29.7305339059327));
#38360=CARTESIAN_POINT('Origin',(9.4,-3.53553390593274,30.0355339059327));
#38361=CARTESIAN_POINT('',(8.685,-3.53553390593274,29.7305339059327));
#38362=CARTESIAN_POINT('Origin',(8.025,-3.53553390593274,22.9644660940673));
#38363=CARTESIAN_POINT('',(8.,-3.53553390593274,22.6094660940673));
#38364=CARTESIAN_POINT('Origin',(8.,-3.53553390593274,22.9644660940673));
#38365=CARTESIAN_POINT('',(8.05,-3.53553390593274,22.6594660940673));
#38366=CARTESIAN_POINT('',(8.025,-3.53553390593274,22.6344660940673));
#38367=CARTESIAN_POINT('Origin',(8.05,-3.53553390593274,22.9644660940673));
#38368=CARTESIAN_POINT('Origin',(8.,-3.53553390593274,22.9644660940673));
#38369=CARTESIAN_POINT('Origin',(8.685,-3.53553390593274,22.9644660940673));
#38370=CARTESIAN_POINT('',(9.4,-3.53553390593274,22.6594660940673));
#38371=CARTESIAN_POINT('Origin',(9.4,-3.53553390593274,22.9644660940673));
#38372=CARTESIAN_POINT('',(8.685,-3.53553390593274,22.6594660940673));
#38373=CARTESIAN_POINT('Origin',(28.425,4.5,6.175));
#38374=CARTESIAN_POINT('',(28.4,9.4,6.2));
#38375=CARTESIAN_POINT('',(28.45,9.4,6.15));
#38376=CARTESIAN_POINT('',(28.4,9.,6.2));
#38377=CARTESIAN_POINT('',(28.4,4.5,6.2));
#38378=CARTESIAN_POINT('',(28.4,9.,6.2));
#38379=CARTESIAN_POINT('Origin',(29.,9.4,6.175));
#38380=CARTESIAN_POINT('',(29.55,9.4,6.15));
#38381=CARTESIAN_POINT('',(29.6,9.4,6.2));
#38382=CARTESIAN_POINT('',(29.55,9.4,6.15));
#38383=CARTESIAN_POINT('Origin',(29.,9.4,6.2));
#38384=CARTESIAN_POINT('Origin',(29.,9.4,6.15));
#38385=CARTESIAN_POINT('Origin',(29.575,4.7,6.175));
#38386=CARTESIAN_POINT('',(29.6,9.,6.2));
#38387=CARTESIAN_POINT('',(29.55,9.,6.15));
#38388=CARTESIAN_POINT('',(29.6,4.7,6.2));
#38389=CARTESIAN_POINT('',(29.55,4.7,6.15));
#38390=CARTESIAN_POINT('Origin',(29.,9.,6.175));
#38391=CARTESIAN_POINT('Origin',(29.,9.,6.2));
#38392=CARTESIAN_POINT('Origin',(29.,9.4,6.2));
#38393=CARTESIAN_POINT('',(29.55,9.4,6.2));
#38394=CARTESIAN_POINT('Origin',(20.,0.,6.2));
#38395=CARTESIAN_POINT('',(30.6999999999995,-10.6423370590827,6.2));
#38396=CARTESIAN_POINT('',(30.665,-10.6784357007116,6.2));
#38397=CARTESIAN_POINT('Ctrl Pts',(30.6999999999992,-10.6423370590825,6.2));
#38398=CARTESIAN_POINT('Ctrl Pts',(30.6883703751711,-10.6549106729719,6.2));
#38399=CARTESIAN_POINT('Ctrl Pts',(30.6767224654731,-10.6669453862552,6.2));
#38400=CARTESIAN_POINT('Ctrl Pts',(30.665,-10.6784357007116,6.2));
#38401=CARTESIAN_POINT('',(30.7,-8.,6.2));
#38402=CARTESIAN_POINT('',(30.7,0.,6.2));
#38403=CARTESIAN_POINT('',(10.05,-8.,6.2));
#38404=CARTESIAN_POINT('',(10.,-8.,6.2));
#38405=CARTESIAN_POINT('',(10.,-7.94827338858625,6.2));
#38406=CARTESIAN_POINT('',(9.57006962784493,-7.50349656267753,6.2));
#38407=CARTESIAN_POINT('',(10.,-4.55,6.2));
#38408=CARTESIAN_POINT('',(10.,-4.5,6.2));
#38409=CARTESIAN_POINT('',(10.05,-4.5,6.2));
#38410=CARTESIAN_POINT('',(13.65,-0.900000000000021,6.2));
#38411=CARTESIAN_POINT('',(30.7,-4.5,6.2));
#38412=CARTESIAN_POINT('',(10.,-4.5,6.2));
#38413=CARTESIAN_POINT('',(30.7,4.5,6.2));
#38414=CARTESIAN_POINT('',(30.7,0.,6.2));
#38415=CARTESIAN_POINT('',(10.,4.5,6.2));
#38416=CARTESIAN_POINT('',(10.05,8.,6.2));
#38417=CARTESIAN_POINT('',(10.1197528260391,8.07216154655071,6.2));
#38418=CARTESIAN_POINT('',(30.7,8.,6.2));
#38419=CARTESIAN_POINT('',(10.,8.,6.2));
#38420=CARTESIAN_POINT('',(30.6999999999995,10.6423370590827,6.2));
#38421=CARTESIAN_POINT('',(30.7,0.,6.2));
#38422=CARTESIAN_POINT('',(30.665,10.6784357007116,6.2));
#38423=CARTESIAN_POINT('Ctrl Pts',(30.665,10.6784357007116,6.2));
#38424=CARTESIAN_POINT('Ctrl Pts',(30.6767224654731,10.6669453862552,6.2));
#38425=CARTESIAN_POINT('Ctrl Pts',(30.6883703751711,10.6549106729719,6.2));
#38426=CARTESIAN_POINT('Ctrl Pts',(30.6999999999992,10.6423370590825,6.2));
#38427=CARTESIAN_POINT('',(30.,10.95,6.2));
#38428=CARTESIAN_POINT('Origin',(30.,10.,6.2));
#38429=CARTESIAN_POINT('',(10.,10.95,6.2));
#38430=CARTESIAN_POINT('',(25.,10.95,6.2));
#38431=CARTESIAN_POINT('',(9.05,10.,6.2));
#38432=CARTESIAN_POINT('Origin',(10.,10.,6.2));
#38433=CARTESIAN_POINT('',(9.05,-10.,6.2));
#38434=CARTESIAN_POINT('',(9.05,5.,6.2));
#38435=CARTESIAN_POINT('',(10.,-10.95,6.2));
#38436=CARTESIAN_POINT('Origin',(10.,-10.,6.2));
#38437=CARTESIAN_POINT('',(30.,-10.95,6.2));
#38438=CARTESIAN_POINT('',(15.,-10.95,6.2));
#38439=CARTESIAN_POINT('Origin',(30.,-10.,6.2));
#38440=CARTESIAN_POINT('',(10.4,-9.,6.2));
#38441=CARTESIAN_POINT('',(10.4,-9.4,6.2));
#38442=CARTESIAN_POINT('',(10.4,-4.7,6.2));
#38443=CARTESIAN_POINT('',(11.6,-9.,6.2));
#38444=CARTESIAN_POINT('Origin',(11.,-9.,6.2));
#38445=CARTESIAN_POINT('',(11.6,-9.4,6.2));
#38446=CARTESIAN_POINT('',(11.6,-4.5,6.2));
#38447=CARTESIAN_POINT('Origin',(11.,-9.4,6.2));
#38448=CARTESIAN_POINT('',(28.4,-9.,6.2));
#38449=CARTESIAN_POINT('',(28.4,-9.4,6.2));
#38450=CARTESIAN_POINT('',(28.4,-4.7,6.2));
#38451=CARTESIAN_POINT('',(29.6,-9.,6.2));
#38452=CARTESIAN_POINT('Origin',(29.,-9.,6.2));
#38453=CARTESIAN_POINT('',(29.6,-9.4,6.2));
#38454=CARTESIAN_POINT('',(29.6,-4.5,6.2));
#38455=CARTESIAN_POINT('Origin',(29.,-9.4,6.2));
#38456=CARTESIAN_POINT('',(10.4,9.4,6.2));
#38457=CARTESIAN_POINT('',(10.4,9.,6.2));
#38458=CARTESIAN_POINT('',(10.4,4.5,6.2));
#38459=CARTESIAN_POINT('',(11.6,9.4,6.2));
#38460=CARTESIAN_POINT('Origin',(11.,9.4,6.2));
#38461=CARTESIAN_POINT('',(11.6,9.,6.2));
#38462=CARTESIAN_POINT('',(11.6,4.7,6.2));
#38463=CARTESIAN_POINT('Origin',(11.,9.,6.2));
#38464=CARTESIAN_POINT('Origin',(10.425,-4.7,6.175));
#38465=CARTESIAN_POINT('',(10.45,-9.,6.15));
#38466=CARTESIAN_POINT('',(10.4,-9.4,6.2));
#38467=CARTESIAN_POINT('Origin',(11.,-9.,6.175));
#38468=CARTESIAN_POINT('',(11.55,-9.,6.15));
#38469=CARTESIAN_POINT('',(11.55,-9.,6.15));
#38470=CARTESIAN_POINT('Origin',(11.,-9.,6.15));
#38471=CARTESIAN_POINT('Origin',(11.575,-4.5,6.175));
#38472=CARTESIAN_POINT('',(11.55,-9.4,6.15));
#38473=CARTESIAN_POINT('',(11.55,-4.5,6.15));
#38474=CARTESIAN_POINT('Origin',(11.,-9.4,6.175));
#38475=CARTESIAN_POINT('Origin',(11.,-9.,6.2));
#38476=CARTESIAN_POINT('',(11.55,-9.,6.2));
#38477=CARTESIAN_POINT('Origin',(10.425,4.5,6.175));
#38478=CARTESIAN_POINT('',(10.45,9.4,6.15));
#38479=CARTESIAN_POINT('',(10.4,9.,6.2));
#38480=CARTESIAN_POINT('Origin',(11.,9.4,6.175));
#38481=CARTESIAN_POINT('',(11.55,9.4,6.15));
#38482=CARTESIAN_POINT('',(11.55,9.4,6.15));
#38483=CARTESIAN_POINT('Origin',(11.,9.4,6.15));
#38484=CARTESIAN_POINT('Origin',(11.575,4.7,6.175));
#38485=CARTESIAN_POINT('',(11.55,9.,6.15));
#38486=CARTESIAN_POINT('',(11.55,4.7,6.15));
#38487=CARTESIAN_POINT('Origin',(11.,9.,6.175));
#38488=CARTESIAN_POINT('Origin',(11.,9.4,6.2));
#38489=CARTESIAN_POINT('',(11.55,9.4,6.2));
#38490=CARTESIAN_POINT('Origin',(28.425,-4.7,6.175));
#38491=CARTESIAN_POINT('',(28.45,-9.,6.15));
#38492=CARTESIAN_POINT('',(28.4,-9.4,6.2));
#38493=CARTESIAN_POINT('Origin',(29.,-9.,6.175));
#38494=CARTESIAN_POINT('',(29.55,-9.,6.15));
#38495=CARTESIAN_POINT('',(29.55,-9.,6.15));
#38496=CARTESIAN_POINT('Origin',(29.,-9.,6.15));
#38497=CARTESIAN_POINT('Origin',(29.575,-4.5,6.175));
#38498=CARTESIAN_POINT('',(29.55,-9.4,6.15));
#38499=CARTESIAN_POINT('',(29.55,-4.5,6.15));
#38500=CARTESIAN_POINT('Origin',(29.,-9.4,6.175));
#38501=CARTESIAN_POINT('Origin',(29.,-9.,6.2));
#38502=CARTESIAN_POINT('',(29.55,-9.,6.2));
#38503=CARTESIAN_POINT('Ctrl Pts',(30.9967839207979,-9.97611773894901,5.94380986596425));
#38504=CARTESIAN_POINT('Ctrl Pts',(30.9968735332431,-9.97499738060725,5.94320279876029));
#38505=CARTESIAN_POINT('Ctrl Pts',(30.9972890756224,-9.9705803344265,5.94081795655504));
#38506=CARTESIAN_POINT('Ctrl Pts',(30.9987938608894,-9.94698237002212,5.92798567506077));
#38507=CARTESIAN_POINT('Ctrl Pts',(30.9996652546658,-9.92505107393448,5.91596719019954));
#38508=CARTESIAN_POINT('Ctrl Pts',(31.0000630673885,-9.90147072833049,5.90303515049092));
#38509=CARTESIAN_POINT('Ctrl Pts',(31.,-9.89703879482902,5.90061245162622));
#38510=CARTESIAN_POINT('Ctrl Pts',(31.,-9.89591670002669,5.9));
#38511=CARTESIAN_POINT('Ctrl Pts',(30.9977590812902,-9.99211390732443,5.91460515238299));
#38512=CARTESIAN_POINT('Ctrl Pts',(30.9978069161407,-9.99125420879031,5.91413815597096));
#38513=CARTESIAN_POINT('Ctrl Pts',(30.9980732319381,-9.98842826990598,5.91261689806809));
#38514=CARTESIAN_POINT('Ctrl Pts',(30.999321009672,-9.96926387849275,5.90220348853136));
#38515=CARTESIAN_POINT('Ctrl Pts',(30.9998924434135,-9.95345363247024,5.89352772308427));
#38516=CARTESIAN_POINT('Ctrl Pts',(31.0001048667676,-9.93430897921292,5.88301910115843));
#38517=CARTESIAN_POINT('Ctrl Pts',(31.,-9.93147133203902,5.88146680533134));
#38518=CARTESIAN_POINT('Ctrl Pts',(31.,-9.93061113335113,5.88099707624835));
#38519=CARTESIAN_POINT('Ctrl Pts',(30.9987342417825,-10.0081100756998,5.88540043880173));
#38520=CARTESIAN_POINT('Ctrl Pts',(30.9987548737402,-10.0075123659462,5.88507472775089));
#38521=CARTESIAN_POINT('Ctrl Pts',(30.9989180472781,-10.0045931974246,5.88348145728224));
#38522=CARTESIAN_POINT('Ctrl Pts',(30.9993345295876,-9.99306004052342,5.87717591947565));
#38523=CARTESIAN_POINT('Ctrl Pts',(30.9997836739084,-9.98034680751244,5.8702235696389));
#38524=CARTESIAN_POINT('Ctrl Pts',(30.9999536075356,-9.96882546804112,5.86391936825949));
#38525=CARTESIAN_POINT('Ctrl Pts',(31.,-9.96590386924902,5.86232115903647));
#38526=CARTESIAN_POINT('Ctrl Pts',(31.,-9.96530556667556,5.8619941524967));
#38527=CARTESIAN_POINT('Ctrl Pts',(30.9997094022748,-10.0241062440753,5.85619572522048));
#38528=CARTESIAN_POINT('Ctrl Pts',(30.9997175112483,-10.0237699570528,5.85601147966085));
#38529=CARTESIAN_POINT('Ctrl Pts',(30.9997551934488,-10.0224437131072,5.85528478208135));
#38530=CARTESIAN_POINT('Ctrl Pts',(30.9998913609518,-10.0153494616369,5.8513983439133));
#38531=CARTESIAN_POINT('Ctrl Pts',(30.999969787671,-10.0087556517074,5.84778686339001));
#38532=CARTESIAN_POINT('Ctrl Pts',(31.000005693946,-10.0016661590036,5.84390391661895));
#38533=CARTESIAN_POINT('Ctrl Pts',(31.,-10.000336406459,5.84317551274159));
#38534=CARTESIAN_POINT('Ctrl Pts',(31.,-10.,5.84299122874504));
#38535=CARTESIAN_POINT('',(30.9967839207979,-9.97611773894901,5.94380986596425));
#38536=CARTESIAN_POINT('Ctrl Pts',(31.,-9.89591670002669,5.9));
#38537=CARTESIAN_POINT('Ctrl Pts',(31.,-9.89628582891983,5.90020147459058));
#38538=CARTESIAN_POINT('Ctrl Pts',(30.999999833778,-9.89665895570928,5.90040514179247));
#38539=CARTESIAN_POINT('Ctrl Pts',(30.9999992763601,-9.89712339088896,5.90065892594312));
#38540=CARTESIAN_POINT('Ctrl Pts',(30.9999986903024,-9.89761168848563,5.90092574937998));
#38541=CARTESIAN_POINT('Ctrl Pts',(30.9999976784015,-9.89820065116803,5.90124782620294));
#38542=CARTESIAN_POINT('Ctrl Pts',(30.9999954463192,-9.89894085089812,5.90165293306493));
#38543=CARTESIAN_POINT('Ctrl Pts',(30.9999930609434,-9.89973188558847,5.90208586159504));
#38544=CARTESIAN_POINT('Ctrl Pts',(30.9999892731396,-9.90069527159664,5.90261341361232));
#38545=CARTESIAN_POINT('Ctrl Pts',(30.9999824925249,-9.90184085130876,5.90324101505058));
#38546=CARTESIAN_POINT('Ctrl Pts',(30.9999749254477,-9.90311930326004,5.90394141003391));
#38547=CARTESIAN_POINT('Ctrl Pts',(30.9999635671848,-9.90462412305264,5.9047661147155));
#38548=CARTESIAN_POINT('Ctrl Pts',(30.9999459978991,-9.9063130903906,5.90569195435123));
#38549=CARTESIAN_POINT('Ctrl Pts',(30.9999225298142,-9.90856912000303,5.90692863998015));
#38550=CARTESIAN_POINT('Ctrl Pts',(30.9998876385962,-9.91115223536192,5.90834496729864));
#38551=CARTESIAN_POINT('Ctrl Pts',(30.9998386164076,-9.91387679834281,5.9098389080064));
#38552=CARTESIAN_POINT('Ctrl Pts',(30.9997947529335,-9.91631464947568,5.91117563799665));
#38553=CARTESIAN_POINT('Ctrl Pts',(30.9997396715424,-9.91886066572249,5.91257171207271));
#38554=CARTESIAN_POINT('Ctrl Pts',(30.9996752373026,-9.92138435056691,5.91395536268362));
#38555=CARTESIAN_POINT('Ctrl Pts',(30.9996230683389,-9.92342764344206,5.91507563070807));
#38556=CARTESIAN_POINT('Ctrl Pts',(30.9995649295049,-9.92545543660446,5.91618728468542));
#38557=CARTESIAN_POINT('Ctrl Pts',(30.9995025257403,-9.92743003826348,5.91726954183405));
#38558=CARTESIAN_POINT('Ctrl Pts',(30.9994457779765,-9.92922567077687,5.91825370798981));
#38559=CARTESIAN_POINT('Ctrl Pts',(30.999385596974,-9.93097685281939,5.91921331456944));
#38560=CARTESIAN_POINT('Ctrl Pts',(30.9993223246179,-9.93269240748663,5.92015306391949));
#38561=CARTESIAN_POINT('Ctrl Pts',(30.9992408992974,-9.93490015818756,5.92136242922035));
#38562=CARTESIAN_POINT('Ctrl Pts',(30.9991545307602,-9.93705010559649,5.92253957558285));
#38563=CARTESIAN_POINT('Ctrl Pts',(30.9990586997045,-9.93925628042519,5.92374645512596));
#38564=CARTESIAN_POINT('Ctrl Pts',(30.9989827215795,-9.94100541097352,5.92470331033505));
#38565=CARTESIAN_POINT('Ctrl Pts',(30.9989006040821,-9.94279114085914,5.92567953304286));
#38566=CARTESIAN_POINT('Ctrl Pts',(30.9988112465986,-9.94462324232011,5.92668030933487));
#38567=CARTESIAN_POINT('Ctrl Pts',(30.9987116641645,-9.94666498651151,5.92779560192353));
#38568=CARTESIAN_POINT('Ctrl Pts',(30.9986030068889,-9.94876376320262,5.92894107424351));
#38569=CARTESIAN_POINT('Ctrl Pts',(30.9984868228399,-9.95087710858715,5.93009346425666));
#38570=CARTESIAN_POINT('Ctrl Pts',(30.9983246628225,-9.95382674002892,5.9317018742406));
#38571=CARTESIAN_POINT('Ctrl Pts',(30.9981474716006,-9.95680342456077,5.93332297948874));
#38572=CARTESIAN_POINT('Ctrl Pts',(30.9979699769605,-9.95959391161321,5.93484096482843));
#38573=CARTESIAN_POINT('Ctrl Pts',(30.9978227927092,-9.96190787302162,5.93609972698306));
#38574=CARTESIAN_POINT('Ctrl Pts',(30.9976759093371,-9.96408899229249,5.93728499112343));
#38575=CARTESIAN_POINT('Ctrl Pts',(30.9975408287681,-9.96601982372525,5.93833347383131));
#38576=CARTESIAN_POINT('Ctrl Pts',(30.9974308421475,-9.9675919641583,5.9391871796652));
#38577=CARTESIAN_POINT('Ctrl Pts',(30.9973288512699,-9.96899745226107,5.93994983139551));
#38578=CARTESIAN_POINT('Ctrl Pts',(30.9972396036754,-9.97020199451459,5.94060317730052));
#38579=CARTESIAN_POINT('Ctrl Pts',(30.9971564144503,-9.97132476916394,5.94121217230859));
#38580=CARTESIAN_POINT('Ctrl Pts',(30.9970843875899,-9.97227236442104,5.94172588660037));
#38581=CARTESIAN_POINT('Ctrl Pts',(30.9970242908726,-9.97305368650373,5.94214938471251));
#38582=CARTESIAN_POINT('Ctrl Pts',(30.9969678010577,-9.97378811496787,5.9425474651904));
#38583=CARTESIAN_POINT('Ctrl Pts',(30.9969218859903,-9.97437530434443,5.94286565959656));
#38584=CARTESIAN_POINT('Ctrl Pts',(30.9968835373317,-9.97486243255521,5.94312963321655));
#38585=CARTESIAN_POINT('Ctrl Pts',(30.9968451886732,-9.97534956076599,5.94339360683654));
#38586=CARTESIAN_POINT('Ctrl Pts',(30.996814458702,-9.9757359460458,5.94360299112644));
#38587=CARTESIAN_POINT('Ctrl Pts',(30.9967839207979,-9.97611773894901,5.94380986596425));
#38588=CARTESIAN_POINT('Ctrl Pts',(30.9997094022748,-10.0241062440753,5.85619572522048));
#38589=CARTESIAN_POINT('Ctrl Pts',(30.9987342417825,-10.0081100756998,5.88540043880173));
#38590=CARTESIAN_POINT('Ctrl Pts',(30.9977590812902,-9.99211390732443,5.91460515238299));
#38591=CARTESIAN_POINT('Ctrl Pts',(30.9967839207979,-9.97611773894901,5.94380986596425));
#38592=CARTESIAN_POINT('Ctrl Pts',(30.9997094013184,10.0241062837382,5.85619574695114));
#38593=CARTESIAN_POINT('Ctrl Pts',(30.9997175103186,10.0237699961624,5.85601150108837));
#38594=CARTESIAN_POINT('Ctrl Pts',(30.9997551926432,10.0224437500347,5.85528480231412));
#38595=CARTESIAN_POINT('Ctrl Pts',(30.9998913605943,10.0153494868895,5.851398357763));
#38596=CARTESIAN_POINT('Ctrl Pts',(30.9999697875716,10.0087556661136,5.84778687129035));
#38597=CARTESIAN_POINT('Ctrl Pts',(31.0000056939647,10.0016661617464,5.84390391812109));
#38598=CARTESIAN_POINT('Ctrl Pts',(31.,10.0003364070128,5.84317551304497));
#38599=CARTESIAN_POINT('Ctrl Pts',(31.,10.,5.84299122874504));
#38600=CARTESIAN_POINT('Ctrl Pts',(30.9987342400859,10.008110115381,5.8854004604625));
#38601=CARTESIAN_POINT('Ctrl Pts',(30.9987548720843,10.0075124050725,5.8850747491106));
#38602=CARTESIAN_POINT('Ctrl Pts',(30.9988790936942,10.0045934168424,5.88348147745615));
#38603=CARTESIAN_POINT('Ctrl Pts',(30.9992674936025,9.99306545616,5.87717593328547));
#38604=CARTESIAN_POINT('Ctrl Pts',(30.9996846877919,9.98035159735118,5.87022357752267));
#38605=CARTESIAN_POINT('Ctrl Pts',(30.9999513575747,9.96882758392452,5.86391936975968));
#38606=CARTESIAN_POINT('Ctrl Pts',(31.,9.96590386980433,5.8623211593403));
#38607=CARTESIAN_POINT('Ctrl Pts',(31.,9.96530556667556,5.8619941524967));
#38608=CARTESIAN_POINT('Ctrl Pts',(30.9977590788535,9.9921139470237,5.91460517397386));
#38609=CARTESIAN_POINT('Ctrl Pts',(30.9978069137501,9.99125424793223,5.91413817726242));
#38610=CARTESIAN_POINT('Ctrl Pts',(30.9981152685796,9.98842830684885,5.91260201951091));
#38611=CARTESIAN_POINT('Ctrl Pts',(30.998967089605,9.96926390369661,5.90207109306701));
#38612=CARTESIAN_POINT('Ctrl Pts',(30.999722710576,9.95345364685531,5.89343987431005));
#38613=CARTESIAN_POINT('Ctrl Pts',(30.9999328116104,9.93430898196904,5.88298760002662));
#38614=CARTESIAN_POINT('Ctrl Pts',(31.,9.93147133259584,5.88146680563563));
#38615=CARTESIAN_POINT('Ctrl Pts',(31.,9.93061113335113,5.88099707624835));
#38616=CARTESIAN_POINT('Ctrl Pts',(30.9967839176211,9.97611777866644,5.94380988748522));
#38617=CARTESIAN_POINT('Ctrl Pts',(30.9968735301548,9.97499741976691,5.94320281998623));
#38618=CARTESIAN_POINT('Ctrl Pts',(30.9972890729406,9.97058037138577,5.94081797664114));
#38619=CARTESIAN_POINT('Ctrl Pts',(30.9987938596804,9.94698239524001,5.92798568903476));
#38620=CARTESIAN_POINT('Ctrl Pts',(30.9996652543314,9.92505108832951,5.91596719818983));
#38621=CARTESIAN_POINT('Ctrl Pts',(31.0000630674513,9.90147073109231,5.90303515199838));
#38622=CARTESIAN_POINT('Ctrl Pts',(31.,9.89703879538735,5.90061245193096));
#38623=CARTESIAN_POINT('Ctrl Pts',(31.,9.89591670002669,5.9));
#38624=CARTESIAN_POINT('',(30.9997094013184,10.0241062837382,5.85619574695114));
#38625=CARTESIAN_POINT('Ctrl Pts',(31.,10.,5.84299122874504));
#38626=CARTESIAN_POINT('Ctrl Pts',(31.,10.0001511918942,5.84307405190661));
#38627=CARTESIAN_POINT('Ctrl Pts',(30.9999999772324,10.0003064637474,5.8431591096781));
#38628=CARTESIAN_POINT('Ctrl Pts',(30.999999861436,10.0005264293687,5.84327959945591));
#38629=CARTESIAN_POINT('Ctrl Pts',(30.9999997332202,10.0007699868055,5.84341301203768));
#38630=CARTESIAN_POINT('Ctrl Pts',(30.9999994934254,10.0010926374677,5.84358974299168));
#38631=CARTESIAN_POINT('Ctrl Pts',(30.9999988482408,10.001517734162,5.84382258165775));
#38632=CARTESIAN_POINT('Ctrl Pts',(30.9999981093085,10.0020045990926,5.84408925270587));
#38633=CARTESIAN_POINT('Ctrl Pts',(30.9999968157179,10.0026250445202,5.8444290830952));
#38634=CARTESIAN_POINT('Ctrl Pts',(30.9999943962796,10.0033477469247,5.84482491679361));
#38635=CARTESIAN_POINT('Ctrl Pts',(30.9999912614642,10.0042841372279,5.84533779019007));
#38636=CARTESIAN_POINT('Ctrl Pts',(30.9999861247826,10.0053880993547,5.84594243788284));
#38637=CARTESIAN_POINT('Ctrl Pts',(30.9999787442318,10.006520052495,5.84656241544142));
#38638=CARTESIAN_POINT('Ctrl Pts',(30.9999728168381,10.007429135317,5.84706032558318));
#38639=CARTESIAN_POINT('Ctrl Pts',(30.9999655108804,10.0083525487905,5.84756608417289));
#38640=CARTESIAN_POINT('Ctrl Pts',(30.9999573082866,10.0092402166771,5.84805226739278));
#38641=CARTESIAN_POINT('Ctrl Pts',(30.9999505378773,10.0099728964872,5.84845356233046));
#38642=CARTESIAN_POINT('Ctrl Pts',(30.9999431973787,10.010680793641,5.84884128535465));
#38643=CARTESIAN_POINT('Ctrl Pts',(30.999935340759,10.0113716446136,5.84921967705076));
#38644=CARTESIAN_POINT('Ctrl Pts',(30.9999270907856,10.0120970840919,5.84961701350323));
#38645=CARTESIAN_POINT('Ctrl Pts',(30.9999182331384,10.0128091746617,5.85000704445293));
#38646=CARTESIAN_POINT('Ctrl Pts',(30.9999082037282,10.0135493216438,5.85041245473004));
#38647=CARTESIAN_POINT('Ctrl Pts',(30.9998975951077,10.0143322129912,5.85084127793111));
#38648=CARTESIAN_POINT('Ctrl Pts',(30.999885633187,10.0151464182939,5.85128726641096));
#38649=CARTESIAN_POINT('Ctrl Pts',(30.9998723269432,10.0159790429398,5.85174335999862));
#38650=CARTESIAN_POINT('Ctrl Pts',(30.9998546101357,10.0170876541093,5.85235063297346));
#38651=CARTESIAN_POINT('Ctrl Pts',(30.9998344254974,10.0182268187928,5.85297467101968));
#38652=CARTESIAN_POINT('Ctrl Pts',(30.9998142545149,10.0192732059832,5.85354790811658));
#38653=CARTESIAN_POINT('Ctrl Pts',(30.9997978064791,10.020126462085,5.85401534316856));
#38654=CARTESIAN_POINT('Ctrl Pts',(30.9997815001227,10.0209137965484,5.85444668062929));
#38655=CARTESIAN_POINT('Ctrl Pts',(30.9997672737566,10.0215730926237,5.85480788085582));
#38656=CARTESIAN_POINT('Ctrl Pts',(30.9997549692658,10.0221433227436,5.85512028564048));
#38657=CARTESIAN_POINT('Ctrl Pts',(30.9997442782914,10.02261667411,5.85537962133272));
#38658=CARTESIAN_POINT('Ctrl Pts',(30.9997358041127,10.022985255601,5.85558155824545));
#38659=CARTESIAN_POINT('Ctrl Pts',(30.9997282393264,10.0233142833877,5.85576182463725));
#38660=CARTESIAN_POINT('Ctrl Pts',(30.9997224549186,10.023559497923,5.85589617331858));
#38661=CARTESIAN_POINT('Ctrl Pts',(30.9997178979514,10.0237513055548,5.85600126110009));
#38662=CARTESIAN_POINT('Ctrl Pts',(30.9997146623179,10.0238874968375,5.85607587773361));
#38663=CARTESIAN_POINT('Ctrl Pts',(30.9997120255593,10.0239974540913,5.85613612116171));
#38664=CARTESIAN_POINT('Ctrl Pts',(30.9997094013184,10.0241062837382,5.85619574695114));
#38665=CARTESIAN_POINT('',(30.9967839176211,9.97611777866644,5.94380988748522));
#38666=CARTESIAN_POINT('Ctrl Pts',(30.9967839176211,9.97611777866644,5.94380988748522));
#38667=CARTESIAN_POINT('Ctrl Pts',(30.9977590788535,9.9921139470237,5.91460517397386));
#38668=CARTESIAN_POINT('Ctrl Pts',(30.9987342400859,10.008110115381,5.8854004604625));
#38669=CARTESIAN_POINT('Ctrl Pts',(30.9997094013184,10.0241062837382,5.85619574695114));
#38670=CARTESIAN_POINT('Ctrl Pts',(30.9967839176211,9.97611777866644,5.94380988748522));
#38671=CARTESIAN_POINT('Ctrl Pts',(30.9968134018443,9.97574915933943,5.94361015076422));
#38672=CARTESIAN_POINT('Ctrl Pts',(30.9968430401383,9.97537653919476,5.94340822589068));
#38673=CARTESIAN_POINT('Ctrl Pts',(30.9968795901821,9.97491255559319,5.94315679475268));
#38674=CARTESIAN_POINT('Ctrl Pts',(30.9969180186502,9.97442472638109,5.94289244175932));
#38675=CARTESIAN_POINT('Ctrl Pts',(30.9969640726959,9.9738361687824,5.94257350817652));
#38676=CARTESIAN_POINT('Ctrl Pts',(30.9970210134522,9.9730962847434,5.94217247405404));
#38677=CARTESIAN_POINT('Ctrl Pts',(30.9970818661454,9.97230556928001,5.94174388813345));
#38678=CARTESIAN_POINT('Ctrl Pts',(30.9971551144017,9.97134239280946,5.94122173226927));
#38679=CARTESIAN_POINT('Ctrl Pts',(30.9972399797972,9.97019691789268,5.94060042376811));
#38680=CARTESIAN_POINT('Ctrl Pts',(30.9973346959385,9.96891848204248,5.93990699691933));
#38681=CARTESIAN_POINT('Ctrl Pts',(30.9974437767348,9.96741351252657,5.93909034512013));
#38682=CARTESIAN_POINT('Ctrl Pts',(30.9975614612863,9.96572428712655,5.93817298465127));
#38683=CARTESIAN_POINT('Ctrl Pts',(30.9977187535123,9.96346653944293,5.9369468791987));
#38684=CARTESIAN_POINT('Ctrl Pts',(30.997890960601,9.96088111561884,5.93554161766041));
#38685=CARTESIAN_POINT('Ctrl Pts',(30.9980605279584,9.95815419184684,5.93405762283485));
#38686=CARTESIAN_POINT('Ctrl Pts',(30.9982120464402,9.95571752386853,5.93273158552184));
#38687=CARTESIAN_POINT('Ctrl Pts',(30.9983611461551,9.95317295204375,5.93134545148876));
#38688=CARTESIAN_POINT('Ctrl Pts',(30.9984992420485,9.950650745604,5.92997002663428));
#38689=CARTESIAN_POINT('Ctrl Pts',(30.9986110968974,9.94860780998098,5.92885596063726));
#38690=CARTESIAN_POINT('Ctrl Pts',(30.9987158226232,9.94658040822982,5.92774940674337));
#38691=CARTESIAN_POINT('Ctrl Pts',(30.9988120790596,9.94460617109134,5.92667098438524));
#38692=CARTESIAN_POINT('Ctrl Pts',(30.9988996170218,9.94281075145494,5.92569024066385));
#38693=CARTESIAN_POINT('Ctrl Pts',(30.998980206257,9.94105976594183,5.9247330233031));
#38694=CARTESIAN_POINT('Ctrl Pts',(30.9990548712986,9.93934432696308,5.92379462024413));
#38695=CARTESIAN_POINT('Ctrl Pts',(30.9991509420324,9.937137089442,5.9225871867724));
#38696=CARTESIAN_POINT('Ctrl Pts',(30.9992374788123,9.9349874579584,5.92141023471798));
#38697=CARTESIAN_POINT('Ctrl Pts',(30.9993190367815,9.93278144537767,5.9202018370499));
#38698=CARTESIAN_POINT('Ctrl Pts',(30.9993837070938,9.93103221689773,5.91924365411179));
#38699=CARTESIAN_POINT('Ctrl Pts',(30.9994451550484,9.92924631016809,5.91826502154007));
#38700=CARTESIAN_POINT('Ctrl Pts',(30.9995030320591,9.92741401288569,5.91726075859807));
#38701=CARTESIAN_POINT('Ctrl Pts',(30.9995675372626,9.92537187720048,5.91614148542615));
#38702=CARTESIAN_POINT('Ctrl Pts',(30.9996274779878,9.92327267550311,5.91499067542366));
#38703=CARTESIAN_POINT('Ctrl Pts',(30.999680967104,9.92115893283402,5.91383177340819));
#38704=CARTESIAN_POINT('Ctrl Pts',(30.999755623503,9.91820871740275,5.91221425834385));
#38705=CARTESIAN_POINT('Ctrl Pts',(30.9998172298906,9.91523150762811,5.91058170643131));
#38706=CARTESIAN_POINT('Ctrl Pts',(30.9998634213129,9.91244064827058,5.90905143958214));
#38707=CARTESIAN_POINT('Ctrl Pts',(30.9999017108032,9.91012721913319,5.9077829543368));
#38708=CARTESIAN_POINT('Ctrl Pts',(30.9999295357067,9.90794663757022,5.90658739090527));
#38709=CARTESIAN_POINT('Ctrl Pts',(30.9999490418999,9.90601621618389,5.90552921905091));
#38710=CARTESIAN_POINT('Ctrl Pts',(30.9999649247195,9.90444438029831,5.90466760795109));
#38711=CARTESIAN_POINT('Ctrl Pts',(30.9999754075208,9.90303911622973,5.90389747901719));
#38712=CARTESIAN_POINT('Ctrl Pts',(30.9999825291478,9.9018346606426,5.90323762352747));
#38713=CARTESIAN_POINT('Ctrl Pts',(30.9999891676432,9.90071191538349,5.90262253266759));
#38714=CARTESIAN_POINT('Ctrl Pts',(30.9999929297512,9.89976424545327,5.90210358223555));
#38715=CARTESIAN_POINT('Ctrl Pts',(30.9999953191642,9.89898272703063,5.90167585189123));
#38716=CARTESIAN_POINT('Ctrl Pts',(30.9999975649231,9.8982481943387,5.90127383715666));
#38717=CARTESIAN_POINT('Ctrl Pts',(30.9999986059227,9.89766075970279,5.90095258053825));
#38718=CARTESIAN_POINT('Ctrl Pts',(30.999999215242,9.89717328034114,5.90068618816431));
#38719=CARTESIAN_POINT('Ctrl Pts',(30.9999998245612,9.89668580097949,5.90041979579038));
#38720=CARTESIAN_POINT('Ctrl Pts',(31.,9.89629895748635,5.90020864030589));
#38721=CARTESIAN_POINT('Ctrl Pts',(31.,9.89591670002669,5.9));
#38722=CARTESIAN_POINT('Ctrl Pts',(30.9967839176211,9.97611777866644,5.94380988748522));
#38723=CARTESIAN_POINT('Ctrl Pts',(30.9917066333316,10.0395952901576,5.97820523540357));
#38724=CARTESIAN_POINT('Ctrl Pts',(30.9741529037903,10.1426508202057,6.03285941899933));
#38725=CARTESIAN_POINT('Ctrl Pts',(30.9167083241675,10.3130060581232,6.11306762286303));
#38726=CARTESIAN_POINT('Ctrl Pts',(30.8426027988904,10.4638132796915,6.17352191726238));
#38727=CARTESIAN_POINT('Ctrl Pts',(30.7487057189956,10.5896778448846,6.20000000000012));
#38728=CARTESIAN_POINT('Ctrl Pts',(30.6999999999992,10.6423370590825,6.2));
#38729=CARTESIAN_POINT('Ctrl Pts',(30.9977590788535,9.9921139470237,5.91460517397386));
#38730=CARTESIAN_POINT('Ctrl Pts',(30.9938642295286,10.055582164711,5.94912303971441));
#38731=CARTESIAN_POINT('Ctrl Pts',(30.978201146713,10.1584856199577,6.00440333149542));
#38732=CARTESIAN_POINT('Ctrl Pts',(30.9236435535527,10.3281478102022,6.08691292609801));
#38733=CARTESIAN_POINT('Ctrl Pts',(30.8518449662238,10.4779872265877,6.15042656152703));
#38734=CARTESIAN_POINT('Ctrl Pts',(30.7594406852812,10.6026091261344,6.18071804878039));
#38735=CARTESIAN_POINT('Ctrl Pts',(30.7112855175703,10.6546595286716,6.18264100709771));
#38736=CARTESIAN_POINT('Ctrl Pts',(30.9987342400859,10.008110115381,5.8854004604625));
#38737=CARTESIAN_POINT('Ctrl Pts',(30.9960218257256,10.0715690392644,5.92004084402524));
#38738=CARTESIAN_POINT('Ctrl Pts',(30.9822493896356,10.1743204197098,5.97594724399151));
#38739=CARTESIAN_POINT('Ctrl Pts',(30.9305787829379,10.3432895622813,6.06075822933298));
#38740=CARTESIAN_POINT('Ctrl Pts',(30.8610871335572,10.4921611734839,6.12733120579168));
#38741=CARTESIAN_POINT('Ctrl Pts',(30.7701756515669,10.6155404073841,6.16143609756066));
#38742=CARTESIAN_POINT('Ctrl Pts',(30.7225710351414,10.6669819982608,6.16528201419542));
#38743=CARTESIAN_POINT('Ctrl Pts',(30.9997094013184,10.0241062837382,5.85619574695114));
#38744=CARTESIAN_POINT('Ctrl Pts',(30.9981794219226,10.0875559138178,5.89095864833608));
#38745=CARTESIAN_POINT('Ctrl Pts',(30.9862976325583,10.1901552194618,5.94749115648761));
#38746=CARTESIAN_POINT('Ctrl Pts',(30.937514012323,10.3584313143604,6.03460353256796));
#38747=CARTESIAN_POINT('Ctrl Pts',(30.8703293008906,10.5063351203802,6.10423585005633));
#38748=CARTESIAN_POINT('Ctrl Pts',(30.7809106178525,10.6284716886339,6.14215414634093));
#38749=CARTESIAN_POINT('Ctrl Pts',(30.7338565527125,10.6793044678499,6.14792302129313));
#38750=CARTESIAN_POINT('',(30.7338565527125,10.6793044678499,6.14792302129313));
#38751=CARTESIAN_POINT('Ctrl Pts',(30.9997094013184,10.0241062837382,5.85619574695114));
#38752=CARTESIAN_POINT('Ctrl Pts',(30.9981794219226,10.0875559138178,5.89095864833608));
#38753=CARTESIAN_POINT('Ctrl Pts',(30.9862976325583,10.1901552194618,5.94749115648761));
#38754=CARTESIAN_POINT('Ctrl Pts',(30.937514012323,10.3584313143604,6.03460353256796));
#38755=CARTESIAN_POINT('Ctrl Pts',(30.8703293008906,10.5063351203802,6.10423585005633));
#38756=CARTESIAN_POINT('Ctrl Pts',(30.7809106178525,10.6284716886339,6.14215414634093));
#38757=CARTESIAN_POINT('Ctrl Pts',(30.7338565527125,10.6793044678499,6.14792302129313));
#38758=CARTESIAN_POINT('',(30.7338565527125,10.6793044678499,6.14792302129313));
#38759=CARTESIAN_POINT('Ctrl Pts',(30.6999999999992,10.6423370590825,6.2));
#38760=CARTESIAN_POINT('Ctrl Pts',(30.7487057189956,10.5896778448846,6.20000000000012));
#38761=CARTESIAN_POINT('Ctrl Pts',(30.8426027988904,10.4638132796915,6.17352191726238));
#38762=CARTESIAN_POINT('Ctrl Pts',(30.9167083241675,10.3130060581232,6.11306762286303));
#38763=CARTESIAN_POINT('Ctrl Pts',(30.9741529037903,10.1426508202057,6.03285941899933));
#38764=CARTESIAN_POINT('Ctrl Pts',(30.9917066333316,10.0395952901576,5.97820523540357));
#38765=CARTESIAN_POINT('Ctrl Pts',(30.9967839176211,9.97611777866644,5.94380988748522));
#38766=CARTESIAN_POINT('Origin',(30.,10.,6.175));
#38767=CARTESIAN_POINT('',(30.,11.,6.15));
#38768=CARTESIAN_POINT('',(30.,11.,6.15));
#38769=CARTESIAN_POINT('',(30.7,10.7141428428543,6.15));
#38770=CARTESIAN_POINT('',(30.665,10.6784357007116,6.2));
#38771=CARTESIAN_POINT('Origin',(30.,10.,6.15));
#38772=CARTESIAN_POINT('Origin',(25.,10.975,6.175));
#38773=CARTESIAN_POINT('',(10.,11.,6.15));
#38774=CARTESIAN_POINT('',(10.,11.,6.15));
#38775=CARTESIAN_POINT('',(25.,11.,6.15));
#38776=CARTESIAN_POINT('Origin',(10.,10.,6.175));
#38777=CARTESIAN_POINT('',(9.,10.,6.15));
#38778=CARTESIAN_POINT('',(9.,10.,6.15));
#38779=CARTESIAN_POINT('Origin',(10.,10.,6.15));
#38780=CARTESIAN_POINT('Origin',(9.025,5.,6.175));
#38781=CARTESIAN_POINT('',(9.,-10.,6.15));
#38782=CARTESIAN_POINT('',(9.,-10.,6.15));
#38783=CARTESIAN_POINT('',(9.,5.,6.15));
#38784=CARTESIAN_POINT('Origin',(10.,-10.,6.175));
#38785=CARTESIAN_POINT('',(10.,-11.,6.15));
#38786=CARTESIAN_POINT('Origin',(10.,-10.,6.15));
#38787=CARTESIAN_POINT('Origin',(15.,-10.975,6.175));
#38788=CARTESIAN_POINT('',(30.,-11.,6.15));
#38789=CARTESIAN_POINT('Origin',(30.,-10.,6.175));
#38790=CARTESIAN_POINT('',(30.7,-10.7141428428543,6.15));
#38791=CARTESIAN_POINT('Ctrl Pts',(30.6999999999992,10.6423370590825,6.2));
#38792=CARTESIAN_POINT('Ctrl Pts',(30.6883703751711,10.6549106729719,6.2));
#38793=CARTESIAN_POINT('Ctrl Pts',(30.6767224654731,10.6669453862552,6.2));
#38794=CARTESIAN_POINT('Ctrl Pts',(30.665,10.6784357007116,6.2));
#38795=CARTESIAN_POINT('Ctrl Pts',(30.7112855175703,10.6546595286716,6.18264100709771));
#38796=CARTESIAN_POINT('Ctrl Pts',(30.6997873496846,10.6670877745971,6.18310015818412));
#38797=CARTESIAN_POINT('Ctrl Pts',(30.6882451720374,10.6789888760943,6.18333333333333));
#38798=CARTESIAN_POINT('Ctrl Pts',(30.6766666666667,10.6903380814258,6.18333333333333));
#38799=CARTESIAN_POINT('Ctrl Pts',(30.7225710351414,10.6669819982608,6.16528201419542));
#38800=CARTESIAN_POINT('Ctrl Pts',(30.7112043241981,10.6792648762223,6.16620031636824));
#38801=CARTESIAN_POINT('Ctrl Pts',(30.6997678786018,10.6910323659335,6.16666666666667));
#38802=CARTESIAN_POINT('Ctrl Pts',(30.6883333333333,10.70224046214,6.16666666666667));
#38803=CARTESIAN_POINT('Ctrl Pts',(30.7338565527125,10.6793044678499,6.14792302129313));
#38804=CARTESIAN_POINT('Ctrl Pts',(30.7226212987117,10.6914419778475,6.14930047455236));
#38805=CARTESIAN_POINT('Ctrl Pts',(30.7112905851662,10.7030758557726,6.15));
#38806=CARTESIAN_POINT('Ctrl Pts',(30.7,10.7141428428543,6.15));
#38807=CARTESIAN_POINT('Ctrl Pts',(30.7338565527125,10.6793044678499,6.14792302129313));
#38808=CARTESIAN_POINT('Ctrl Pts',(30.7226212987117,10.6914419778475,6.14930047455236));
#38809=CARTESIAN_POINT('Ctrl Pts',(30.7112905851662,10.7030758557726,6.15));
#38810=CARTESIAN_POINT('Ctrl Pts',(30.7,10.7141428428543,6.15));
#38811=CARTESIAN_POINT('Ctrl Pts',(30.6999999999992,-10.6423370590825,6.2));
#38812=CARTESIAN_POINT('Ctrl Pts',(30.7293995132925,-10.6105511559129,6.20000000000007));
#38813=CARTESIAN_POINT('Ctrl Pts',(30.7582382311623,-10.5755441820079,6.19560373930292));
#38814=CARTESIAN_POINT('Ctrl Pts',(30.8178826904194,-10.4935177749275,6.17800728102166));
#38815=CARTESIAN_POINT('Ctrl Pts',(30.8614297222427,-10.4226084466948,6.15570478058127));
#38816=CARTESIAN_POINT('Ctrl Pts',(30.9162763309817,-10.3099389124345,6.11112745456547));
#38817=CARTESIAN_POINT('Ctrl Pts',(30.9447582561879,-10.2331375716414,6.07591295728));
#38818=CARTESIAN_POINT('Ctrl Pts',(30.9792320402833,-10.1123553378356,6.01669471341596));
#38819=CARTESIAN_POINT('Ctrl Pts',(30.9915707246235,-10.0412944876546,5.97912594754713));
#38820=CARTESIAN_POINT('Ctrl Pts',(30.9967839207979,-9.97611773894901,5.94380986596425));
#38821=CARTESIAN_POINT('Ctrl Pts',(30.7112855175703,-10.6546595286716,6.18264100709771));
#38822=CARTESIAN_POINT('Ctrl Pts',(30.7403530419617,-10.6232428387308,6.1814758827751));
#38823=CARTESIAN_POINT('Ctrl Pts',(30.7688042988717,-10.5886067472929,6.17593248602285));
#38824=CARTESIAN_POINT('Ctrl Pts',(30.8274420633668,-10.5073652408122,6.15590971324675));
#38825=CARTESIAN_POINT('Ctrl Pts',(30.8700216323188,-10.437031263705,6.13182321060776));
#38826=CARTESIAN_POINT('Ctrl Pts',(30.9231458705104,-10.3250728058919,6.08499529598356));
#38827=CARTESIAN_POINT('Ctrl Pts',(30.9503483536313,-10.2486255880964,6.04862265724997));
#38828=CARTESIAN_POINT('Ctrl Pts',(30.9827269941712,-10.1282330114988,5.98806638775668));
#38829=CARTESIAN_POINT('Ctrl Pts',(30.9937578217055,-10.0572879383963,5.95003794609275));
#38830=CARTESIAN_POINT('Ctrl Pts',(30.9977590812902,-9.99211390732443,5.91460515238299));
#38831=CARTESIAN_POINT('Ctrl Pts',(30.7225710351414,-10.6669819982608,6.16528201419542));
#38832=CARTESIAN_POINT('Ctrl Pts',(30.7513055739305,-10.635929345816,6.16296495779396));
#38833=CARTESIAN_POINT('Ctrl Pts',(30.7793686753514,-10.6016729290708,6.15625008908845));
#38834=CARTESIAN_POINT('Ctrl Pts',(30.837003966094,-10.5212046804115,6.13383250447826));
#38835=CARTESIAN_POINT('Ctrl Pts',(30.878614593152,-10.45144908405,6.10795182991645));
#38836=CARTESIAN_POINT('Ctrl Pts',(30.9300172225282,-10.3402007573639,6.05887633762058));
#38837=CARTESIAN_POINT('Ctrl Pts',(30.955947099261,-10.2641021226664,6.02135776304424));
#38838=CARTESIAN_POINT('Ctrl Pts',(30.9862108563741,-10.1441174667834,5.95941345010241));
#38839=CARTESIAN_POINT('Ctrl Pts',(30.9959513738211,-10.0732608461654,5.92097716308504));
#38840=CARTESIAN_POINT('Ctrl Pts',(30.9987342417825,-10.0081100756998,5.88540043880173));
#38841=CARTESIAN_POINT('Ctrl Pts',(30.7338565527125,-10.6793044678499,6.14792302129313));
#38842=CARTESIAN_POINT('Ctrl Pts',(30.7622591025997,-10.6486210286339,6.14444084056899));
#38843=CARTESIAN_POINT('Ctrl Pts',(30.7899347430608,-10.6147354943559,6.13657883580837));
#38844=CARTESIAN_POINT('Ctrl Pts',(30.8465633390414,-10.5350521462962,6.11173493670335));
#38845=CARTESIAN_POINT('Ctrl Pts',(30.8872065032282,-10.4658719010602,6.08407025994295));
#38846=CARTESIAN_POINT('Ctrl Pts',(30.9368867620569,-10.3553346508213,6.03274417903868));
#38847=CARTESIAN_POINT('Ctrl Pts',(30.9615371967044,-10.2795901391215,5.99406746301422));
#38848=CARTESIAN_POINT('Ctrl Pts',(30.989705810262,-10.1599951404466,5.93078512444313));
#38849=CARTESIAN_POINT('Ctrl Pts',(30.9981384709031,-10.0892542969071,5.89188916163067));
#38850=CARTESIAN_POINT('Ctrl Pts',(30.9997094022748,-10.0241062440753,5.85619572522048));
#38851=CARTESIAN_POINT('Ctrl Pts',(30.9967839207979,-9.97611773894901,5.94380986596425));
#38852=CARTESIAN_POINT('Ctrl Pts',(30.9915707246235,-10.0412944876546,5.97912594754713));
#38853=CARTESIAN_POINT('Ctrl Pts',(30.9792320402833,-10.1123553378356,6.01669471341596));
#38854=CARTESIAN_POINT('Ctrl Pts',(30.9447582561879,-10.2331375716414,6.07591295728));
#38855=CARTESIAN_POINT('Ctrl Pts',(30.9162763309817,-10.3099389124345,6.11112745456547));
#38856=CARTESIAN_POINT('Ctrl Pts',(30.8614297222427,-10.4226084466948,6.15570478058127));
#38857=CARTESIAN_POINT('Ctrl Pts',(30.8178826904194,-10.4935177749275,6.17800728102166));
#38858=CARTESIAN_POINT('Ctrl Pts',(30.7582382311623,-10.5755441820079,6.19560373930292));
#38859=CARTESIAN_POINT('Ctrl Pts',(30.7293995132925,-10.6105511559129,6.20000000000007));
#38860=CARTESIAN_POINT('Ctrl Pts',(30.6999999999992,-10.6423370590825,6.2));
#38861=CARTESIAN_POINT('',(30.6999999999995,-10.6423370590827,6.2));
#38862=CARTESIAN_POINT('Ctrl Pts',(30.665,-10.6784357007116,6.2));
#38863=CARTESIAN_POINT('Ctrl Pts',(30.6767224654731,-10.6669453862552,6.2));
#38864=CARTESIAN_POINT('Ctrl Pts',(30.6883703751711,-10.6549106729719,6.2));
#38865=CARTESIAN_POINT('Ctrl Pts',(30.6999999999992,-10.6423370590825,6.2));
#38866=CARTESIAN_POINT('Ctrl Pts',(30.6766666666667,-10.6903380814258,6.18333333333333));
#38867=CARTESIAN_POINT('Ctrl Pts',(30.6882451720374,-10.6789888760944,6.18333333333333));
#38868=CARTESIAN_POINT('Ctrl Pts',(30.6997873496846,-10.6670877745971,6.18310015818412));
#38869=CARTESIAN_POINT('Ctrl Pts',(30.7112855175703,-10.6546595286716,6.18264100709771));
#38870=CARTESIAN_POINT('Ctrl Pts',(30.6883333333333,-10.70224046214,6.16666666666667));
#38871=CARTESIAN_POINT('Ctrl Pts',(30.6997678786018,-10.6910323659335,6.16666666666667));
#38872=CARTESIAN_POINT('Ctrl Pts',(30.7112043241981,-10.6792648762223,6.16620031636824));
#38873=CARTESIAN_POINT('Ctrl Pts',(30.7225710351414,-10.6669819982608,6.16528201419542));
#38874=CARTESIAN_POINT('Ctrl Pts',(30.7,-10.7141428428543,6.15));
#38875=CARTESIAN_POINT('Ctrl Pts',(30.7112905851662,-10.7030758557726,6.15));
#38876=CARTESIAN_POINT('Ctrl Pts',(30.7226212987117,-10.6914419778475,6.14930047455236));
#38877=CARTESIAN_POINT('Ctrl Pts',(30.7338565527125,-10.6793044678499,6.14792302129313));
#38878=CARTESIAN_POINT('Origin',(30.7,0.,5.9));
#38879=CARTESIAN_POINT('Origin',(30.7,-7.76915840380663,5.9));
#38880=CARTESIAN_POINT('Origin',(10.,-10.,4.2));
#38881=CARTESIAN_POINT('',(9.,-10.,4.2));
#38882=CARTESIAN_POINT('Origin',(9.,10.,4.2));
#38883=CARTESIAN_POINT('',(9.,10.,4.2));
#38884=CARTESIAN_POINT('Origin',(10.,10.,4.2));
#38885=CARTESIAN_POINT('',(10.,11.,4.2));
#38886=CARTESIAN_POINT('Origin',(30.,11.,4.2));
#38887=CARTESIAN_POINT('',(30.,11.,4.2));
#38888=CARTESIAN_POINT('Origin',(10.025,-4.525,10.35));
#38889=CARTESIAN_POINT('',(10.05,-4.5,8.95830089865305));
#38890=CARTESIAN_POINT('',(10.05,-4.5,10.35));
#38891=CARTESIAN_POINT('',(10.,-4.55,8.96086067249887));
#38892=CARTESIAN_POINT('',(10.,-4.55,10.35));
#38893=CARTESIAN_POINT('Ctrl Pts',(10.,-4.55,8.96086067249887));
#38894=CARTESIAN_POINT('Ctrl Pts',(10.0166666720695,-4.53333332793054,8.96000796626512));
#38895=CARTESIAN_POINT('Ctrl Pts',(10.0333333561696,-4.51666664383039,8.95915470813818));
#38896=CARTESIAN_POINT('Ctrl Pts',(10.05,-4.5,8.95830089865305));
#38897=CARTESIAN_POINT('Origin',(29.2841674687199,-4.525,6.98243503368624));
#38898=CARTESIAN_POINT('',(11.2135541721682,-4.55,14.));
#38899=CARTESIAN_POINT('Origin',(29.2841674687199,-4.55,6.98243503368624));
#38900=CARTESIAN_POINT('',(11.2601630224385,-4.5,13.9818998597663));
#38901=CARTESIAN_POINT('',(11.2135541721682,-4.55,14.));
#38902=CARTESIAN_POINT('Origin',(29.2841674687199,-4.5,6.98243503368624));
#38903=CARTESIAN_POINT('Ctrl Pts',(11.2672025025441,-4.5,14.));
#38904=CARTESIAN_POINT('Ctrl Pts',(11.391959999534,-4.5,14.3203062297749));
#38905=CARTESIAN_POINT('Ctrl Pts',(11.668054446774,-4.4303581677262,14.9774819072439));
#38906=CARTESIAN_POINT('Ctrl Pts',(12.1316598081387,-4.10683395243209,15.9286468865022));
#38907=CARTESIAN_POINT('Ctrl Pts',(12.524997260418,-3.67159465412862,16.6376752255481));
#38908=CARTESIAN_POINT('Ctrl Pts',(12.8177228984641,-3.24811960222038,17.1263128398011));
#38909=CARTESIAN_POINT('Ctrl Pts',(13.0898330833522,-2.78494101931705,17.5607918840079));
#38910=CARTESIAN_POINT('Ctrl Pts',(13.4127915844491,-2.06816050302593,18.0433746309751));
#38911=CARTESIAN_POINT('Ctrl Pts',(13.6504781966751,-1.17371806751399,18.3757567399041));
#38912=CARTESIAN_POINT('Ctrl Pts',(13.7448250712003,-0.34677769024255,18.5049230225636));
#38913=CARTESIAN_POINT('Ctrl Pts',(13.7445858103348,0.346816939957277,18.5045458836767));
#38914=CARTESIAN_POINT('Ctrl Pts',(13.6373623529499,1.29192272955491,18.3578766190094));
#38915=CARTESIAN_POINT('Ctrl Pts',(13.3722017145503,2.17594495900127,17.9861325476814));
#38916=CARTESIAN_POINT('Ctrl Pts',(13.0443130403164,2.86199680217774,17.4880641812068));
#38917=CARTESIAN_POINT('Ctrl Pts',(12.8178440847237,3.24806162865946,17.1265367900342));
#38918=CARTESIAN_POINT('Ctrl Pts',(12.5249752388355,3.67157303457683,16.6376360062934));
#38919=CARTESIAN_POINT('Ctrl Pts',(12.1317232805211,4.10675982821366,15.928729275166));
#38920=CARTESIAN_POINT('Ctrl Pts',(11.6680306338885,4.43037992268562,14.9774496711636));
#38921=CARTESIAN_POINT('Ctrl Pts',(11.391959999534,4.5,14.3203062297749));
#38922=CARTESIAN_POINT('Ctrl Pts',(11.2672025025441,4.5,14.));
#38923=CARTESIAN_POINT('Ctrl Pts',(11.2516950047624,-4.51665435240168,14.006107294649));
#38924=CARTESIAN_POINT('Ctrl Pts',(11.3769625715924,-4.51621852393914,14.3277191173693));
#38925=CARTESIAN_POINT('Ctrl Pts',(11.6541843464077,-4.44533549720252,14.9873034081241));
#38926=CARTESIAN_POINT('Ctrl Pts',(12.119584202532,-4.119207886609,15.9409930517025));
#38927=CARTESIAN_POINT('Ctrl Pts',(12.5143327076105,-3.68158280890167,16.6511544706723));
#38928=CARTESIAN_POINT('Ctrl Pts',(12.8080550666115,-3.25627951505913,17.1402234548367));
#38929=CARTESIAN_POINT('Ctrl Pts',(13.0810645349093,-2.79136044400086,17.5748911978179));
#38930=CARTESIAN_POINT('Ctrl Pts',(13.405044673385,-2.07240378878844,18.0573316981621));
#38931=CARTESIAN_POINT('Ctrl Pts',(13.6434562871566,-1.17593865460604,18.3893328785638));
#38932=CARTESIAN_POINT('Ctrl Pts',(13.7380888018818,-0.347413383593392,
18.5183095858136));
#38933=CARTESIAN_POINT('Ctrl Pts',(13.7378488054313,0.347453340477631,18.5179320837059));
#38934=CARTESIAN_POINT('Ctrl Pts',(13.6303006408794,1.29436558132429,18.3714809661723));
#38935=CARTESIAN_POINT('Ctrl Pts',(13.364330921006,2.18046915754007,18.0001463863418));
#38936=CARTESIAN_POINT('Ctrl Pts',(13.035394038305,2.86870807689454,17.5021311417631));
#38937=CARTESIAN_POINT('Ctrl Pts',(12.8081766935965,3.25622047982334,17.1404479014005));
#38938=CARTESIAN_POINT('Ctrl Pts',(12.5143106100714,3.68156157484352,16.6511151239475));
#38939=CARTESIAN_POINT('Ctrl Pts',(12.1196478076241,4.11913346993114,15.9410753393783));
#38940=CARTESIAN_POINT('Ctrl Pts',(11.6541604800616,4.44535739714532,14.9872711896631));
#38941=CARTESIAN_POINT('Ctrl Pts',(11.3769625715924,4.51621852393914,14.3277191173693));
#38942=CARTESIAN_POINT('Ctrl Pts',(11.2516950047624,4.51665435240168,14.0061072946491));
#38943=CARTESIAN_POINT('Ctrl Pts',(11.2361875069806,-4.53330870480335,14.0122145892981));
#38944=CARTESIAN_POINT('Ctrl Pts',(11.3619651436507,-4.53243704787828,14.3351320049637));
#38945=CARTESIAN_POINT('Ctrl Pts',(11.6403142460414,-4.46031282667885,14.9971249090043));
#38946=CARTESIAN_POINT('Ctrl Pts',(12.1075085969253,-4.1315818207859,15.9533392169029));
#38947=CARTESIAN_POINT('Ctrl Pts',(12.503668154803,-3.69157096367473,16.6646337157966));
#38948=CARTESIAN_POINT('Ctrl Pts',(12.798387234759,-3.26443942789788,17.1541340698723));
#38949=CARTESIAN_POINT('Ctrl Pts',(13.0722959864663,-2.79777986868466,17.588990511628));
#38950=CARTESIAN_POINT('Ctrl Pts',(13.3972977623209,-2.07664707455095,18.071288765349));
#38951=CARTESIAN_POINT('Ctrl Pts',(13.6364343776382,-1.1781592416981,18.4029090172236));
#38952=CARTESIAN_POINT('Ctrl Pts',(13.7313525325633,-0.348049076944234,
18.5316961490636));
#38953=CARTESIAN_POINT('Ctrl Pts',(13.7311118005278,0.348089740997986,18.5313182837351));
#38954=CARTESIAN_POINT('Ctrl Pts',(13.6232389288088,1.29680843309367,18.3850853133351));
#38955=CARTESIAN_POINT('Ctrl Pts',(13.3564601274617,2.18499335607887,18.0141602250022));
#38956=CARTESIAN_POINT('Ctrl Pts',(13.0264750362935,2.87541935161135,17.5161981023194));
#38957=CARTESIAN_POINT('Ctrl Pts',(12.7985093024693,3.26437933098722,17.1543590127667));
#38958=CARTESIAN_POINT('Ctrl Pts',(12.5036459813074,3.6915501151102,16.6645942416017));
#38959=CARTESIAN_POINT('Ctrl Pts',(12.1075723347271,4.13150711164862,15.9534214035907));
#38960=CARTESIAN_POINT('Ctrl Pts',(11.6402903262347,4.46033487160503,14.9970927081627));
#38961=CARTESIAN_POINT('Ctrl Pts',(11.3619651436507,4.53243704787828,14.3351320049637));
#38962=CARTESIAN_POINT('Ctrl Pts',(11.2361875069806,4.53330870480335,14.0122145892981));
#38963=CARTESIAN_POINT('Ctrl Pts',(11.2206800091989,-4.54996305720503,14.0183218839471));
#38964=CARTESIAN_POINT('Ctrl Pts',(11.346967715709,-4.54865557181743,14.342544892558));
#38965=CARTESIAN_POINT('Ctrl Pts',(11.6264441456752,-4.47529015615518,15.0069464098845));
#38966=CARTESIAN_POINT('Ctrl Pts',(12.0954329913186,-4.14395575496281,15.9656853821032));
#38967=CARTESIAN_POINT('Ctrl Pts',(12.4930036019956,-3.70155911844778,16.6781129609208));
#38968=CARTESIAN_POINT('Ctrl Pts',(12.7887194029065,-3.27259934073663,17.1680446849079));
#38969=CARTESIAN_POINT('Ctrl Pts',(13.0635274380233,-2.80419929336847,17.6030898254381));
#38970=CARTESIAN_POINT('Ctrl Pts',(13.3895508512568,-2.08089036031346,18.0852458325359));
#38971=CARTESIAN_POINT('Ctrl Pts',(13.6294124681197,-1.18037982879015,18.4164851558833));
#38972=CARTESIAN_POINT('Ctrl Pts',(13.7246162632449,-0.348684770295076,
18.5450827123137));
#38973=CARTESIAN_POINT('Ctrl Pts',(13.7243747956243,0.34872614151834,18.5447044837643));
#38974=CARTESIAN_POINT('Ctrl Pts',(13.6161772167383,1.29925128486305,18.3986896604979));
#38975=CARTESIAN_POINT('Ctrl Pts',(13.3485893339173,2.18951755461767,18.0281740636625));
#38976=CARTESIAN_POINT('Ctrl Pts',(13.017556034282,2.88213062632815,17.5302650628756));
#38977=CARTESIAN_POINT('Ctrl Pts',(12.7888419113421,3.2725381821511,17.168270124133));
#38978=CARTESIAN_POINT('Ctrl Pts',(12.4929813525433,3.70153865537689,16.6780733592558));
#38979=CARTESIAN_POINT('Ctrl Pts',(12.0954968618301,4.14388075336609,15.965767467803));
#38980=CARTESIAN_POINT('Ctrl Pts',(11.6264201724079,4.47531234606473,15.0069142266622));
#38981=CARTESIAN_POINT('Ctrl Pts',(11.3469677157091,4.54865557181743,14.342544892558));
#38982=CARTESIAN_POINT('Ctrl Pts',(11.2206800091989,4.54996305720503,14.0183218839471));
#38983=CARTESIAN_POINT('',(11.2672025025441,-4.5,14.));
#38984=CARTESIAN_POINT('',(11.2206800091989,-4.54996305720503,14.0183218839471));
#38985=CARTESIAN_POINT('',(11.2672025025441,-4.5,14.));
#38986=CARTESIAN_POINT('',(11.2206800091989,4.54996305720503,14.0183218839471));
#38987=CARTESIAN_POINT('Ctrl Pts',(11.2206800091989,-4.54996305720503,14.0183218839471));
#38988=CARTESIAN_POINT('Ctrl Pts',(11.346967715709,-4.54865557181743,14.342544892558));
#38989=CARTESIAN_POINT('Ctrl Pts',(11.6264441456752,-4.47529015615518,15.0069464098845));
#38990=CARTESIAN_POINT('Ctrl Pts',(12.0954329913186,-4.14395575496281,15.9656853821032));
#38991=CARTESIAN_POINT('Ctrl Pts',(12.4930036019956,-3.70155911844778,16.6781129609208));
#38992=CARTESIAN_POINT('Ctrl Pts',(12.7887194029065,-3.27259934073663,17.1680446849079));
#38993=CARTESIAN_POINT('Ctrl Pts',(13.0635274380233,-2.80419929336847,17.6030898254381));
#38994=CARTESIAN_POINT('Ctrl Pts',(13.3895508512568,-2.08089036031346,18.0852458325359));
#38995=CARTESIAN_POINT('Ctrl Pts',(13.6294124681197,-1.18037982879015,18.4164851558833));
#38996=CARTESIAN_POINT('Ctrl Pts',(13.7246162632449,-0.348684770295076,
18.5450827123137));
#38997=CARTESIAN_POINT('Ctrl Pts',(13.7243747956243,0.34872614151834,18.5447044837643));
#38998=CARTESIAN_POINT('Ctrl Pts',(13.6161772167383,1.29925128486305,18.3986896604979));
#38999=CARTESIAN_POINT('Ctrl Pts',(13.3485893339173,2.18951755461767,18.0281740636625));
#39000=CARTESIAN_POINT('Ctrl Pts',(13.017556034282,2.88213062632815,17.5302650628756));
#39001=CARTESIAN_POINT('Ctrl Pts',(12.7888419113421,3.2725381821511,17.168270124133));
#39002=CARTESIAN_POINT('Ctrl Pts',(12.4929813525433,3.70153865537689,16.6780733592558));
#39003=CARTESIAN_POINT('Ctrl Pts',(12.0954968618301,4.14388075336609,15.965767467803));
#39004=CARTESIAN_POINT('Ctrl Pts',(11.6264201724079,4.47531234606473,15.0069142266622));
#39005=CARTESIAN_POINT('Ctrl Pts',(11.3469677157091,4.54865557181743,14.342544892558));
#39006=CARTESIAN_POINT('Ctrl Pts',(11.2206800091989,4.54996305720503,14.0183218839471));
#39007=CARTESIAN_POINT('',(11.2672025025441,4.5,14.));
#39008=CARTESIAN_POINT('',(11.2206800091989,4.54996305720503,14.0183218839471));
#39009=CARTESIAN_POINT('Ctrl Pts',(11.2672025025441,4.5,14.));
#39010=CARTESIAN_POINT('Ctrl Pts',(11.391959999534,4.5,14.3203062297749));
#39011=CARTESIAN_POINT('Ctrl Pts',(11.6680306338885,4.43037992268562,14.9774496711636));
#39012=CARTESIAN_POINT('Ctrl Pts',(12.1317232805211,4.10675982821366,15.928729275166));
#39013=CARTESIAN_POINT('Ctrl Pts',(12.5249752388355,3.67157303457683,16.6376360062934));
#39014=CARTESIAN_POINT('Ctrl Pts',(12.8178440847237,3.24806162865946,17.1265367900342));
#39015=CARTESIAN_POINT('Ctrl Pts',(13.0443130403164,2.86199680217774,17.4880641812068));
#39016=CARTESIAN_POINT('Ctrl Pts',(13.3722017145503,2.17594495900127,17.9861325476814));
#39017=CARTESIAN_POINT('Ctrl Pts',(13.6373623529499,1.29192272955491,18.3578766190094));
#39018=CARTESIAN_POINT('Ctrl Pts',(13.7445858103348,0.346816939957277,18.5045458836767));
#39019=CARTESIAN_POINT('Ctrl Pts',(13.7448250712003,-0.34677769024255,18.5049230225636));
#39020=CARTESIAN_POINT('Ctrl Pts',(13.6504781966751,-1.17371806751399,18.3757567399041));
#39021=CARTESIAN_POINT('Ctrl Pts',(13.4127915844491,-2.06816050302593,18.0433746309751));
#39022=CARTESIAN_POINT('Ctrl Pts',(13.0898330833522,-2.78494101931705,17.5607918840079));
#39023=CARTESIAN_POINT('Ctrl Pts',(12.8177228984641,-3.24811960222038,17.1263128398011));
#39024=CARTESIAN_POINT('Ctrl Pts',(12.524997260418,-3.67159465412862,16.6376752255481));
#39025=CARTESIAN_POINT('Ctrl Pts',(12.1316598081387,-4.10683395243209,15.9286468865022));
#39026=CARTESIAN_POINT('Ctrl Pts',(11.668054446774,-4.4303581677262,14.9774819072439));
#39027=CARTESIAN_POINT('Ctrl Pts',(11.391959999534,-4.5,14.3203062297749));
#39028=CARTESIAN_POINT('Ctrl Pts',(11.2672025025441,-4.5,14.));
#39029=CARTESIAN_POINT('Ctrl Pts',(11.2601630224385,-4.5,13.9818998597663));
#39030=CARTESIAN_POINT('Ctrl Pts',(11.2625048863574,-4.5,13.9879302873398));
#39031=CARTESIAN_POINT('Ctrl Pts',(11.2648513789474,-4.5,13.9939636530615));
#39032=CARTESIAN_POINT('Ctrl Pts',(11.2672025025441,-4.5,14.));
#39033=CARTESIAN_POINT('Ctrl Pts',(11.244626739015,-4.51666666666667,13.9879332398442));
#39034=CARTESIAN_POINT('Ctrl Pts',(11.2469781779907,-4.51666666666667,13.9939883237121));
#39035=CARTESIAN_POINT('Ctrl Pts',(11.2493342686192,-4.51666256582858,14.000046343094));
#39036=CARTESIAN_POINT('Ctrl Pts',(11.2516950047624,-4.51665435240168,14.006107294649));
#39037=CARTESIAN_POINT('Ctrl Pts',(11.2290904555916,-4.53333333333333,13.9939666199221));
#39038=CARTESIAN_POINT('Ctrl Pts',(11.2314514696241,-4.53333333333333,14.0000463600845));
#39039=CARTESIAN_POINT('Ctrl Pts',(11.233817158291,-4.53332513165716,14.0061290331264));
#39040=CARTESIAN_POINT('Ctrl Pts',(11.2361875069806,-4.53330870480335,14.0122145892981));
#39041=CARTESIAN_POINT('Ctrl Pts',(11.2135541721682,-4.55,14.));
#39042=CARTESIAN_POINT('Ctrl Pts',(11.2159247612574,-4.55,14.0061043964569));
#39043=CARTESIAN_POINT('Ctrl Pts',(11.2183000479628,-4.54998769748575,14.0122117231589));
#39044=CARTESIAN_POINT('Ctrl Pts',(11.2206800091989,-4.54996305720503,14.0183218839471));
#39045=CARTESIAN_POINT('Ctrl Pts',(11.2672025025441,-4.5,14.));
#39046=CARTESIAN_POINT('Ctrl Pts',(11.2648513789474,-4.5,13.9939636530615));
#39047=CARTESIAN_POINT('Ctrl Pts',(11.2625048863574,-4.5,13.9879302873398));
#39048=CARTESIAN_POINT('Ctrl Pts',(11.2601630224385,-4.5,13.9818998597663));
#39049=CARTESIAN_POINT('Ctrl Pts',(11.2135541721682,-4.55,14.));
#39050=CARTESIAN_POINT('Ctrl Pts',(11.2159247612574,-4.55,14.0061043964569));
#39051=CARTESIAN_POINT('Ctrl Pts',(11.2183000479628,-4.54998769748575,14.0122117231589));
#39052=CARTESIAN_POINT('Ctrl Pts',(11.2206800091989,-4.54996305720503,14.0183218839471));
#39053=CARTESIAN_POINT('Ctrl Pts',(11.2672025025441,4.5,14.));
#39054=CARTESIAN_POINT('Ctrl Pts',(11.2648513789474,4.5,13.9939636530615));
#39055=CARTESIAN_POINT('Ctrl Pts',(11.2625048863574,4.5,13.9879302873398));
#39056=CARTESIAN_POINT('Ctrl Pts',(11.2601630224385,4.5,13.9818998597663));
#39057=CARTESIAN_POINT('Ctrl Pts',(11.2516950047624,4.51665435240168,14.0061072946491));
#39058=CARTESIAN_POINT('Ctrl Pts',(11.2493342686192,4.51666256582858,14.000046343094));
#39059=CARTESIAN_POINT('Ctrl Pts',(11.2469781779907,4.51666666666667,13.9939883237121));
#39060=CARTESIAN_POINT('Ctrl Pts',(11.244626739015,4.51666666666667,13.9879332398442));
#39061=CARTESIAN_POINT('Ctrl Pts',(11.2361875069806,4.53330870480335,14.0122145892981));
#39062=CARTESIAN_POINT('Ctrl Pts',(11.233817158291,4.53332513165716,14.0061290331264));
#39063=CARTESIAN_POINT('Ctrl Pts',(11.2314514696241,4.53333333333333,14.0000463600845));
#39064=CARTESIAN_POINT('Ctrl Pts',(11.2290904555916,4.53333333333333,13.9939666199221));
#39065=CARTESIAN_POINT('Ctrl Pts',(11.2206800091989,4.54996305720503,14.0183218839471));
#39066=CARTESIAN_POINT('Ctrl Pts',(11.2183000479628,4.54998769748575,14.0122117231589));
#39067=CARTESIAN_POINT('Ctrl Pts',(11.2159247612574,4.55,14.0061043964569));
#39068=CARTESIAN_POINT('Ctrl Pts',(11.2135541721682,4.55,14.));
#39069=CARTESIAN_POINT('Ctrl Pts',(11.2601630224385,4.5,13.9818998597663));
#39070=CARTESIAN_POINT('Ctrl Pts',(11.2625048863574,4.5,13.9879302873398));
#39071=CARTESIAN_POINT('Ctrl Pts',(11.2648513789474,4.5,13.9939636530615));
#39072=CARTESIAN_POINT('Ctrl Pts',(11.2672025025441,4.5,14.));
#39073=CARTESIAN_POINT('Ctrl Pts',(11.2206800091989,4.54996305720503,14.0183218839471));
#39074=CARTESIAN_POINT('Ctrl Pts',(11.2183000479628,4.54998769748575,14.0122117231589));
#39075=CARTESIAN_POINT('Ctrl Pts',(11.2159247612574,4.55,14.0061043964569));
#39076=CARTESIAN_POINT('Ctrl Pts',(11.2135541721682,4.55,14.));
#39077=CARTESIAN_POINT('Origin',(10.,-4.5,6.2));
#39078=CARTESIAN_POINT('',(30.7,-4.5,14.));
#39079=CARTESIAN_POINT('',(10.,-4.5,14.));
#39080=CARTESIAN_POINT('',(30.7,-4.5,10.35));
#39081=CARTESIAN_POINT('Origin',(10.,0.,14.));
#39082=CARTESIAN_POINT('',(30.7,4.5,14.));
#39083=CARTESIAN_POINT('',(10.,4.5,14.));
#39084=CARTESIAN_POINT('Origin',(30.7,0.,14.));
#39085=CARTESIAN_POINT('Origin',(10.,4.5,14.));
#39086=CARTESIAN_POINT('',(30.7,4.5,14.25));
#39087=CARTESIAN_POINT('Origin',(10.025,-4.48546421904046,19.3618097929987));
#39088=CARTESIAN_POINT('',(10.,-7.21647899346606,8.96086067249887));
#39089=CARTESIAN_POINT('',(10.,-4.46129870798463,19.3554044768152));
#39090=CARTESIAN_POINT('',(10.05,-7.26883964150479,8.95846862523193));
#39091=CARTESIAN_POINT('',(10.05,-4.5096297300963,19.3682151091821));
#39092=CARTESIAN_POINT('',(10.0000172096761,-7.21645233550652,8.96102841378919));
#39093=CARTESIAN_POINT('Ctrl Pts',(10.0499999997418,-7.26883964123718,8.95846862523692));
#39094=CARTESIAN_POINT('Ctrl Pts',(10.041668961232,-7.26010965815917,8.95888836093242));
#39095=CARTESIAN_POINT('Ctrl Pts',(10.0333384789044,-7.25137933806241,8.95931153454445));
#39096=CARTESIAN_POINT('Ctrl Pts',(10.0250085549945,-7.24264868518276,8.95973813882635));
#39097=CARTESIAN_POINT('Ctrl Pts',(10.0166689007691,-7.23390783388976,8.96016524143145));
#39098=CARTESIAN_POINT('Ctrl Pts',(10.0083297538089,-7.22516658949489,8.96059579976206));
#39099=CARTESIAN_POINT('Ctrl Pts',(10.0000172232168,-7.21645233580055,8.96102841200166));
#39100=CARTESIAN_POINT('Origin',(29.2841674687199,-27.6909737118631,6.98243503368624));
#39101=CARTESIAN_POINT('Ctrl Pts',(17.652334347801,-3.69831792998691,22.4290732641403));
#39102=CARTESIAN_POINT('Ctrl Pts',(16.7444852861922,-3.87955529520026,21.7453141135627));
#39103=CARTESIAN_POINT('Ctrl Pts',(15.0497308464295,-4.28458970814565,20.2172297374505));
#39104=CARTESIAN_POINT('Ctrl Pts',(12.715241047622,-5.08051171703884,17.2144330675353));
#39105=CARTESIAN_POINT('Ctrl Pts',(10.8707604156826,-6.07967020878362,13.4448805759527));
#39106=CARTESIAN_POINT('Ctrl Pts',(10.204866996482,-6.8692113042336,10.4661573522096));
#39107=CARTESIAN_POINT('Ctrl Pts',(10.05,-7.26883964150479,8.95846862523193));
#39108=CARTESIAN_POINT('Ctrl Pts',(17.6399944278817,-3.67849079088921,22.4402019872628));
#39109=CARTESIAN_POINT('Ctrl Pts',(16.7312990590247,-3.85991565088488,21.7556121939904));
#39110=CARTESIAN_POINT('Ctrl Pts',(15.0350589231358,-4.26536148427094,20.225717321171));
#39111=CARTESIAN_POINT('Ctrl Pts',(12.6988460476652,-5.06205511383136,17.2195925305481));
#39112=CARTESIAN_POINT('Ctrl Pts',(10.8534507340507,-6.06212749181112,13.4462167968078));
#39113=CARTESIAN_POINT('Ctrl Pts',(10.1876458579098,-6.85234295886588,10.4648029623686));
#39114=CARTESIAN_POINT('Ctrl Pts',(10.0329820767251,-7.25230186474275,8.95583316773031));
#39115=CARTESIAN_POINT('Ctrl Pts',(17.6276545079625,-3.65866365179151,22.4513307103853));
#39116=CARTESIAN_POINT('Ctrl Pts',(16.7181128318572,-3.8402760065695,21.7659102744182));
#39117=CARTESIAN_POINT('Ctrl Pts',(15.0203869998421,-4.24613326039624,20.2342049048915));
#39118=CARTESIAN_POINT('Ctrl Pts',(12.6824510477084,-5.04359851062388,17.2247519935608));
#39119=CARTESIAN_POINT('Ctrl Pts',(10.8361410524188,-6.04458477483863,13.4475530176629));
#39120=CARTESIAN_POINT('Ctrl Pts',(10.1704247193375,-6.83547461349816,10.4634485725276));
#39121=CARTESIAN_POINT('Ctrl Pts',(10.0159641534501,-7.23576408798071,8.95319771022869));
#39122=CARTESIAN_POINT('Ctrl Pts',(17.6153145880432,-3.63883651269381,22.4624594335078));
#39123=CARTESIAN_POINT('Ctrl Pts',(16.7049266046897,-3.82063636225412,21.776208354846));
#39124=CARTESIAN_POINT('Ctrl Pts',(15.0057150765484,-4.22690503652154,20.242692488612));
#39125=CARTESIAN_POINT('Ctrl Pts',(12.6660560477516,-5.02514190741641,17.2299114565736));
#39126=CARTESIAN_POINT('Ctrl Pts',(10.8188313707869,-6.02704205786613,13.448889238518));
#39127=CARTESIAN_POINT('Ctrl Pts',(10.1532035807653,-6.81860626813044,10.4620941826865));
#39128=CARTESIAN_POINT('Ctrl Pts',(9.99894623017517,-7.21922631121867,8.95056225272706));
#39129=CARTESIAN_POINT('Ctrl Pts',(10.05,-7.26883964150479,8.95846862523193));
#39130=CARTESIAN_POINT('Ctrl Pts',(10.204866996482,-6.8692113042336,10.4661573522096));
#39131=CARTESIAN_POINT('Ctrl Pts',(10.8707604156826,-6.07967020878362,13.4448805759527));
#39132=CARTESIAN_POINT('Ctrl Pts',(12.715241047622,-5.08051171703884,17.2144330675353));
#39133=CARTESIAN_POINT('Ctrl Pts',(15.0497308464295,-4.28458970814565,20.2172297374505));
#39134=CARTESIAN_POINT('Ctrl Pts',(16.7444852861922,-3.87955529520026,21.7453141135627));
#39135=CARTESIAN_POINT('Ctrl Pts',(17.652334347801,-3.69831792998691,22.4290732641403));
#39136=CARTESIAN_POINT('Ctrl Pts',(17.5228110256662,-3.65742470091966,22.3922935453347));
#39137=CARTESIAN_POINT('Ctrl Pts',(16.6473289621003,-3.83444881028949,21.7240714551034));
#39138=CARTESIAN_POINT('Ctrl Pts',(14.9818879132372,-4.23503430666294,20.2120102290229));
#39139=CARTESIAN_POINT('Ctrl Pts',(12.6660560477516,-5.02514190741641,17.2299114565736));
#39140=CARTESIAN_POINT('Ctrl Pts',(10.8203817853331,-6.02620114198486,13.4520627300372));
#39141=CARTESIAN_POINT('Ctrl Pts',(10.1547408409013,-6.81677931654233,10.4689877869414));
#39142=CARTESIAN_POINT('Ctrl Pts',(10.0000172232168,-7.21645233580054,8.96102841200167));
#39143=CARTESIAN_POINT('Origin',(10.,0.,14.5));
#39144=CARTESIAN_POINT('',(10.,0.,8.96086067249887));
#39145=CARTESIAN_POINT('Origin',(29.2841674687199,0.,6.98243503368624));
#39146=CARTESIAN_POINT('',(10.0000172098585,7.21645233533023,8.96102841374249));
#39147=CARTESIAN_POINT('Ctrl Pts',(10.0000172182924,7.21645233578529,8.96102841204531));
#39148=CARTESIAN_POINT('Ctrl Pts',(10.1159693818364,6.91692872721562,10.0911257931426));
#39149=CARTESIAN_POINT('Ctrl Pts',(10.5478144953569,6.32240188608982,12.3343975511604));
#39150=CARTESIAN_POINT('Ctrl Pts',(11.9121133386251,5.37960601026696,15.8921642658605));
#39151=CARTESIAN_POINT('Ctrl Pts',(14.169114976772,4.45071152571792,19.397921706989));
#39152=CARTESIAN_POINT('Ctrl Pts',(16.3452550272053,3.89553380888615,21.4934907341451));
#39153=CARTESIAN_POINT('Ctrl Pts',(17.5228113952696,3.6574248207145,22.3922930928554));
#39154=CARTESIAN_POINT('Origin',(29.2841674687199,27.6909737118635,6.98243503368624));
#39155=CARTESIAN_POINT('Origin',(10.025,6.68546421904046,11.0618097929987));
#39156=CARTESIAN_POINT('',(10.05,7.2688396415048,8.9584686252319));
#39157=CARTESIAN_POINT('',(10.05,6.7096297300963,11.0682151091822));
#39158=CARTESIAN_POINT('Ctrl Pts',(10.0000172182908,7.21645233578921,8.9610284120305));
#39159=CARTESIAN_POINT('Ctrl Pts',(10.0083297493438,7.2251665882511,8.96059579984804));
#39160=CARTESIAN_POINT('Ctrl Pts',(10.0166689056817,7.23390784118624,8.96016524108607));
#39161=CARTESIAN_POINT('Ctrl Pts',(10.0250085688505,7.24264870099244,8.95973813806369));
#39162=CARTESIAN_POINT('Ctrl Pts',(10.0333385064594,7.25137936737065,8.95931153312091));
#39163=CARTESIAN_POINT('Ctrl Pts',(10.0416689753296,7.26010967292925,8.95888836022941));
#39164=CARTESIAN_POINT('Ctrl Pts',(10.0499999999962,7.26883964150102,8.95846862523143));
#39165=CARTESIAN_POINT('Ctrl Pts',(10.05,7.2688396415048,8.9584686252319));
#39166=CARTESIAN_POINT('Ctrl Pts',(10.1661502473615,6.9691183885514,10.0892351704652));
#39167=CARTESIAN_POINT('Ctrl Pts',(10.5984429848576,6.37513989100329,12.3301540475785));
#39168=CARTESIAN_POINT('Ctrl Pts',(11.9625932588821,5.43398809923566,15.8808630801564));
#39169=CARTESIAN_POINT('Ctrl Pts',(14.2362718966461,4.49906819572165,19.4080608979592));
#39170=CARTESIAN_POINT('Ctrl Pts',(16.4418689323227,3.93996775027137,21.5173943967035));
#39171=CARTESIAN_POINT('Ctrl Pts',(17.652334347801,3.69831792998691,22.4290732641403));
#39172=CARTESIAN_POINT('Ctrl Pts',(10.0329820767251,7.25230186474276,8.95583316773028));
#39173=CARTESIAN_POINT('Ctrl Pts',(10.1489799126136,6.9523326853351,10.087560513709));
#39174=CARTESIAN_POINT('Ctrl Pts',(10.5811465692894,6.35785097057932,12.3304726305192));
#39175=CARTESIAN_POINT('Ctrl Pts',(11.9457666187964,5.4158607362461,15.8846301420578));
#39176=CARTESIAN_POINT('Ctrl Pts',(14.2209166065999,4.4800558859075,19.4156012755794));
#39177=CARTESIAN_POINT('Ctrl Pts',(16.4284006027391,3.92039060421677,21.527415596233));
#39178=CARTESIAN_POINT('Ctrl Pts',(17.6399944278817,3.67849079088921,22.4402019872628));
#39179=CARTESIAN_POINT('Ctrl Pts',(10.0159641534501,7.23576408798071,8.95319771022866));
#39180=CARTESIAN_POINT('Ctrl Pts',(10.1318095778657,6.9355469821188,10.0858858569528));
#39181=CARTESIAN_POINT('Ctrl Pts',(10.5638501537211,6.34056205015536,12.3307912134598));
#39182=CARTESIAN_POINT('Ctrl Pts',(11.9289399787108,5.39773337325653,15.8883972039592));
#39183=CARTESIAN_POINT('Ctrl Pts',(14.2055613165538,4.46104357609334,19.4231416531995));
#39184=CARTESIAN_POINT('Ctrl Pts',(16.4149322731554,3.90081345816216,21.5374367957625));
#39185=CARTESIAN_POINT('Ctrl Pts',(17.6276545079625,3.65866365179151,22.4513307103853));
#39186=CARTESIAN_POINT('Ctrl Pts',(9.99894623017517,7.21922631121867,8.95056225272703));
#39187=CARTESIAN_POINT('Ctrl Pts',(10.1146392431178,6.9187612789025,10.0842112001966));
#39188=CARTESIAN_POINT('Ctrl Pts',(10.5465537381528,6.3232731297314,12.3311097964004));
#39189=CARTESIAN_POINT('Ctrl Pts',(11.9121133386251,5.37960601026696,15.8921642658605));
#39190=CARTESIAN_POINT('Ctrl Pts',(14.1902060265076,4.44203126627919,19.4306820308196));
#39191=CARTESIAN_POINT('Ctrl Pts',(16.4014639435718,3.88123631210755,21.5474579952921));
#39192=CARTESIAN_POINT('Ctrl Pts',(17.6153145880432,3.63883651269381,22.4624594335078));
#39193=CARTESIAN_POINT('Ctrl Pts',(17.652334347801,3.69831792998691,22.4290732641403));
#39194=CARTESIAN_POINT('Ctrl Pts',(16.4418689323227,3.93996775027137,21.5173943967035));
#39195=CARTESIAN_POINT('Ctrl Pts',(14.2362718966461,4.49906819572165,19.4080608979592));
#39196=CARTESIAN_POINT('Ctrl Pts',(11.9625932588821,5.43398809923566,15.8808630801564));
#39197=CARTESIAN_POINT('Ctrl Pts',(10.5984429848576,6.37513989100329,12.3301540475785));
#39198=CARTESIAN_POINT('Ctrl Pts',(10.1661502473615,6.9691183885514,10.0892351704652));
#39199=CARTESIAN_POINT('Ctrl Pts',(10.05,7.2688396415048,8.9584686252319));
#39200=CARTESIAN_POINT('Origin',(10.,8.,6.2));
#39201=CARTESIAN_POINT('',(30.7,3.81894289852426,21.9739881555676));
#39202=CARTESIAN_POINT('Ctrl Pts',(30.7,3.81894289852426,21.9739881555676));
#39203=CARTESIAN_POINT('Ctrl Pts',(30.7,3.78282920367073,22.1102352770604));
#39204=CARTESIAN_POINT('Ctrl Pts',(30.7525414730858,3.73863720875327,22.2769596215218));
#39205=CARTESIAN_POINT('Ctrl Pts',(30.8616200595593,3.70421517668381,22.4068245606929));
#39206=CARTESIAN_POINT('Ctrl Pts',(30.883201857851,3.69834545349182,22.4289694254627));
#39207=CARTESIAN_POINT('',(30.7,6.7096297300963,11.0682151091821));
#39208=CARTESIAN_POINT('Origin',(30.7,6.41964359742627,10.9913513149805));
#39209=CARTESIAN_POINT('Origin',(30.7,3.52895676585423,21.8971243613659));
#39210=CARTESIAN_POINT('Origin',(30.7,7.76915840380663,5.9));
#39211=CARTESIAN_POINT('Ctrl Pts',(30.7,3.81894289852426,21.9739881555676));
#39212=CARTESIAN_POINT('Ctrl Pts',(30.7,3.78282920367073,22.1102352770604));
#39213=CARTESIAN_POINT('Ctrl Pts',(30.7715940999863,3.72261227565378,22.3374173236698));
#39214=CARTESIAN_POINT('Ctrl Pts',(31.0187900704284,3.66370490435624,22.5596587699287));
#39215=CARTESIAN_POINT('Ctrl Pts',(31.206032048618,3.65068523769029,22.6087784214412));
#39216=CARTESIAN_POINT('Ctrl Pts',(31.3,3.65068523769029,22.6087784214412));
#39217=CARTESIAN_POINT('Ctrl Pts',(30.7897597901026,3.81894289852426,21.9739881555676));
#39218=CARTESIAN_POINT('Ctrl Pts',(30.7848964349226,3.78727672262178,22.0927550475032));
#39219=CARTESIAN_POINT('Ctrl Pts',(30.8394512775623,3.73340196864192,22.296531662366));
#39220=CARTESIAN_POINT('Ctrl Pts',(31.0522093360623,3.67909470247398,22.5008277705934));
#39221=CARTESIAN_POINT('Ctrl Pts',(31.2172125765626,3.66718808492154,22.5465176796142));
#39222=CARTESIAN_POINT('Ctrl Pts',(31.3,3.66718808492154,22.5465176796142));
#39223=CARTESIAN_POINT('Ctrl Pts',(30.9451341282606,3.74609392831331,21.9546787899695));
#39224=CARTESIAN_POINT('Ctrl Pts',(30.9324919958102,3.73076953859995,22.045697702757));
#39225=CARTESIAN_POINT('Ctrl Pts',(30.9576800464939,3.70077983961214,22.2119544443171));
#39226=CARTESIAN_POINT('Ctrl Pts',(31.1107940637027,3.66738281103999,22.3880924247951));
#39227=CARTESIAN_POINT('Ctrl Pts',(31.2366864832781,3.65961053535241,22.4282347250844));
#39228=CARTESIAN_POINT('Ctrl Pts',(31.3,3.65961053535241,22.4282347250844));
#39229=CARTESIAN_POINT('Ctrl Pts',(31.,3.59402950185702,21.9143725564509));
#39230=CARTESIAN_POINT('Ctrl Pts',(30.9943394443927,3.5941157545723,21.9980577360181));
#39231=CARTESIAN_POINT('Ctrl Pts',(31.0222220993468,3.59316689985222,22.1457612036113));
#39232=CARTESIAN_POINT('Ctrl Pts',(31.1487007374675,3.5918369340252,22.2993482759741));
#39233=CARTESIAN_POINT('Ctrl Pts',(31.2494296143552,3.59144914920715,22.3342075571237));
#39234=CARTESIAN_POINT('Ctrl Pts',(31.3,3.59144914920715,22.3342075571237));
#39235=CARTESIAN_POINT('Ctrl Pts',(31.,3.52895676585423,21.8971243613659));
#39236=CARTESIAN_POINT('Ctrl Pts',(31.,3.53242173859483,21.9817483837486));
#39237=CARTESIAN_POINT('Ctrl Pts',(31.0357970499931,3.54051530807604,22.1255567476876));
#39238=CARTESIAN_POINT('Ctrl Pts',(31.1593950352142,3.55173936013825,22.2704611196166));
#39239=CARTESIAN_POINT('Ctrl Pts',(31.253016024309,3.55458559184835,22.3029866249648));
#39240=CARTESIAN_POINT('Ctrl Pts',(31.3,3.55458559184835,22.3029866249648));
#39241=CARTESIAN_POINT('Ctrl Pts',(31.3,3.55458559184835,22.3029866249648));
#39242=CARTESIAN_POINT('Ctrl Pts',(31.2756424398013,3.55458559184835,22.3029866249648));
#39243=CARTESIAN_POINT('Ctrl Pts',(31.251325303224,3.5542555152723,22.2986589576326));
#39244=CARTESIAN_POINT('Ctrl Pts',(31.2278365577763,3.55358711671133,22.2904495989342));
#39245=CARTESIAN_POINT('Ctrl Pts',(31.21687917868,3.55327531221602,22.2866199752705));
#39246=CARTESIAN_POINT('Ctrl Pts',(31.2061028246701,3.55288981741005,22.2819458574035));
#39247=CARTESIAN_POINT('Ctrl Pts',(31.1955904369623,3.55242800636988,22.2764746103786));
#39248=CARTESIAN_POINT('Ctrl Pts',(31.1851646913517,3.55197000153227,22.27104845685));
#39249=CARTESIAN_POINT('Ctrl Pts',(31.1749846707102,3.55145727885839,22.2648486445406));
#39250=CARTESIAN_POINT('Ctrl Pts',(31.1651324221987,3.55089593171273,22.2579251705824));
#39251=CARTESIAN_POINT('Ctrl Pts',(31.1440506461922,3.54969476481436,22.243110366936));
#39252=CARTESIAN_POINT('Ctrl Pts',(31.1244713735838,3.54827125610268,22.2249790389089));
#39253=CARTESIAN_POINT('Ctrl Pts',(31.1067914803827,3.54673218450983,22.204390880169));
#39254=CARTESIAN_POINT('Ctrl Pts',(31.1039119222156,3.54648151296309,22.2010376472072));
#39255=CARTESIAN_POINT('Ctrl Pts',(31.1010826937327,3.54622776561751,22.1976193381469));
#39256=CARTESIAN_POINT('Ctrl Pts',(31.0983054351552,3.54597138811509,22.1941397675718));
#39257=CARTESIAN_POINT('Ctrl Pts',(31.0849112824948,3.54473493162016,22.1773585071401));
#39258=CARTESIAN_POINT('Ctrl Pts',(31.0726984287011,3.54343307339863,22.159116102809));
#39259=CARTESIAN_POINT('Ctrl Pts',(31.0618470492513,3.54212767814902,22.139817606453));
#39260=CARTESIAN_POINT('Ctrl Pts',(31.0476338473508,3.54041786362005,22.1145403201548));
#39261=CARTESIAN_POINT('Ctrl Pts',(31.0357565901788,3.53870186217841,22.0874512813291));
#39262=CARTESIAN_POINT('Ctrl Pts',(31.0263360245292,3.53705605792282,22.0592732093212));
#39263=CARTESIAN_POINT('Ctrl Pts',(31.0146072529624,3.53500700239098,22.0241910091578));
#39264=CARTESIAN_POINT('Ctrl Pts',(31.0067007874871,3.53305164285664,21.9874657655656));
#39265=CARTESIAN_POINT('Ctrl Pts',(31.0028067335223,3.53130572162164,21.9504036863965));
#39266=CARTESIAN_POINT('Ctrl Pts',(31.0009438970831,3.53047050831289,21.9326739394002));
#39267=CARTESIAN_POINT('Ctrl Pts',(31.,3.52968323549415,21.9148667182822));
#39268=CARTESIAN_POINT('Ctrl Pts',(31.,3.52895676585423,21.8971243613659));
#39269=CARTESIAN_POINT('Ctrl Pts',(31.3,-3.65068523769029,22.6087784214412));
#39270=CARTESIAN_POINT('Ctrl Pts',(31.2060320492444,-3.65068523769029,22.6087784214412));
#39271=CARTESIAN_POINT('Ctrl Pts',(31.0661575833834,-3.66040229491942,22.5721186146222));
#39272=CARTESIAN_POINT('Ctrl Pts',(30.7974922692494,-3.7104074533064,22.3834627897986));
#39273=CARTESIAN_POINT('Ctrl Pts',(30.7,-3.77079130527928,22.1556509846282));
#39274=CARTESIAN_POINT('Ctrl Pts',(30.7,-3.81894289852426,21.9739881555676));
#39275=CARTESIAN_POINT('Ctrl Pts',(31.3,-3.66718808492154,22.5465176796142));
#39276=CARTESIAN_POINT('Ctrl Pts',(31.2172125771145,-3.66718808492154,22.5465176796142));
#39277=CARTESIAN_POINT('Ctrl Pts',(31.0940449626308,-3.67606150627315,22.5124376348801));
#39278=CARTESIAN_POINT('Ctrl Pts',(30.8609238321856,-3.7222672059363,22.3387523169962));
#39279=CARTESIAN_POINT('Ctrl Pts',(30.7832753165149,-3.77672133056048,22.1323440118337));
#39280=CARTESIAN_POINT('Ctrl Pts',(30.7897597901026,-3.81894289852426,21.9739881555676));
#39281=CARTESIAN_POINT('Ctrl Pts',(31.3,-3.65961053535241,22.4282347250844));
#39282=CARTESIAN_POINT('Ctrl Pts',(31.2366864837002,-3.65961053535241,22.4282347250844));
#39283=CARTESIAN_POINT('Ctrl Pts',(31.1429041474226,-3.66539136745645,22.3983436223796));
#39284=CARTESIAN_POINT('Ctrl Pts',(30.9713984134312,-3.69396820322993,22.2480618211276));
#39285=CARTESIAN_POINT('Ctrl Pts',(30.9282779516226,-3.72566140865002,22.0760373406227));
#39286=CARTESIAN_POINT('Ctrl Pts',(30.9451341282606,-3.74609392831331,21.9546787899695));
#39287=CARTESIAN_POINT('Ctrl Pts',(31.3,-3.59144914920716,22.3342075571237));
#39288=CARTESIAN_POINT('Ctrl Pts',(31.2494296146924,-3.59144914920716,22.3342075571237));
#39289=CARTESIAN_POINT('Ctrl Pts',(31.174304730506,-3.59174798363142,22.308273695567));
#39290=CARTESIAN_POINT('Ctrl Pts',(31.0343816236694,-3.59285979234815,22.1772532407699));
#39291=CARTESIAN_POINT('Ctrl Pts',(30.9924525925068,-3.59414450547755,22.025952796122));
#39292=CARTESIAN_POINT('Ctrl Pts',(31.,-3.59402950185703,21.9143725564509));
#39293=CARTESIAN_POINT('Ctrl Pts',(31.3,-3.55458559184835,22.3029866249648));
#39294=CARTESIAN_POINT('Ctrl Pts',(31.2530160246223,-3.55458559184835,22.3029866249648));
#39295=CARTESIAN_POINT('Ctrl Pts',(31.1830787916917,-3.55250612095037,22.2787754248841));
#39296=CARTESIAN_POINT('Ctrl Pts',(31.0487461346247,-3.5426930738467,22.155375588576));
#39297=CARTESIAN_POINT('Ctrl Pts',(31.,-3.53357672951851,22.0099563914605));
#39298=CARTESIAN_POINT('Ctrl Pts',(31.,-3.52895676585423,21.8971243613659));
#39299=CARTESIAN_POINT('',(30.7,-3.81894289852426,21.9739881555676));
#39300=CARTESIAN_POINT('Origin',(30.7,-3.52895676585423,21.8971243613659));
#39301=CARTESIAN_POINT('Ctrl Pts',(31.,-3.52895676585423,21.8971243613659));
#39302=CARTESIAN_POINT('Ctrl Pts',(31.,-3.53357672951851,22.0099563914605));
#39303=CARTESIAN_POINT('Ctrl Pts',(31.0487461346247,-3.5426930738467,22.155375588576));
#39304=CARTESIAN_POINT('Ctrl Pts',(31.1830787916917,-3.55250612095037,22.2787754248841));
#39305=CARTESIAN_POINT('Ctrl Pts',(31.2530160246223,-3.55458559184835,22.3029866249648));
#39306=CARTESIAN_POINT('Ctrl Pts',(31.3,-3.55458559184835,22.3029866249648));
#39307=CARTESIAN_POINT('Ctrl Pts',(30.8832668539234,-3.69836097281072,22.428910875305));
#39308=CARTESIAN_POINT('Ctrl Pts',(30.7656075273914,-3.73048633809753,22.3077106335411));
#39309=CARTESIAN_POINT('Ctrl Pts',(30.7,-3.77478001583655,22.1406026675257));
#39310=CARTESIAN_POINT('Ctrl Pts',(30.7,-3.81894289852426,21.9739881555676));
#39311=CARTESIAN_POINT('Origin',(30.7,-4.21964359742627,19.2913513149805));
#39312=CARTESIAN_POINT('',(30.7,-4.5096297300963,19.3682151091822));
#39313=CARTESIAN_POINT('Origin',(10.,-3.6,22.8));
#39314=CARTESIAN_POINT('Origin',(30.7,-4.8,10.35));
#39315=CARTESIAN_POINT('Origin',(30.7,-4.8,14.));
#39316=CARTESIAN_POINT('Origin',(30.7,-4.8,5.9));
#39317=CARTESIAN_POINT('Origin',(30.7,0.,5.9));
#39318=CARTESIAN_POINT('Origin',(30.7,4.8,5.9));
#39319=CARTESIAN_POINT('Origin',(30.7,0.,14.));
#39320=CARTESIAN_POINT('Origin',(30.7,4.8,14.));
#39321=CARTESIAN_POINT('Origin',(30.7,4.8,14.25));
#39322=CARTESIAN_POINT('Origin',(30.7,0.,5.9));
#39323=CARTESIAN_POINT('Origin',(30.,10.,4.2));
#39324=CARTESIAN_POINT('Origin',(31.3,0.,26.5));
#39325=CARTESIAN_POINT('Origin',(29.55,9.4,6.2));
#39326=CARTESIAN_POINT('Origin',(11.55,-9.,6.2));
#39327=CARTESIAN_POINT('Origin',(11.55,9.4,6.2));
#39328=CARTESIAN_POINT('Origin',(29.55,-9.,6.2));
#39329=CARTESIAN_POINT('Origin',(9.4916312444017,3.53553390593274,22.9644660940673));
#39330=CARTESIAN_POINT('',(9.58326248880341,3.53553390593274,22.9644660940673));
#39331=CARTESIAN_POINT('',(9.4916312444017,3.53553390593274,22.8119660940673));
#39332=CARTESIAN_POINT('Origin',(9.4916312444017,-3.53553390593274,22.9644660940673));
#39333=CARTESIAN_POINT('',(9.58326248880341,-3.53553390593274,22.9644660940673));
#39334=CARTESIAN_POINT('',(9.4916312444017,-3.53553390593274,22.8119660940673));
#39335=CARTESIAN_POINT('Origin',(9.4916312444017,-3.53553390593274,30.0355339059327));
#39336=CARTESIAN_POINT('',(9.58326248880341,-3.53553390593274,30.0355339059327));
#39337=CARTESIAN_POINT('',(9.4916312444017,-3.53553390593274,29.8830339059327));
#39338=CARTESIAN_POINT('Origin',(9.4916312444017,3.53553390593274,30.0355339059327));
#39339=CARTESIAN_POINT('',(9.58326248880341,3.53553390593274,30.0355339059327));
#39340=CARTESIAN_POINT('',(9.4916312444017,3.53553390593274,29.8830339059327));
#39341=CARTESIAN_POINT('Origin',(34.905,0.,21.2));
#39342=CARTESIAN_POINT('',(34.095,-4.95981953654679E-17,21.2));
#39343=CARTESIAN_POINT('Origin',(34.5,0.,21.2));
#39344=CARTESIAN_POINT('Origin',(34.5,0.,22.4));
#39345=CARTESIAN_POINT('',(34.095,-5.94935672022701E-17,23.));
#39346=CARTESIAN_POINT('',(34.095,-4.95981953654679E-17,22.4));
#39347=CARTESIAN_POINT('',(34.5,-0.405000000000001,23.0235111103298));
#39348=CARTESIAN_POINT('Ctrl Pts',(34.5,-0.405000000000001,23.0235111103298));
#39349=CARTESIAN_POINT('Ctrl Pts',(34.449098166481,-0.405000000000001,23.0235111103298));
#39350=CARTESIAN_POINT('Ctrl Pts',(34.3948349045423,-0.39481791137655,23.0222778822844));
#39351=CARTESIAN_POINT('Ctrl Pts',(34.2950649266667,-0.353472062708214,
23.0178325988594));
#39352=CARTESIAN_POINT('Ctrl Pts',(34.2495542896821,-0.322310782443173,
23.0146857230619));
#39353=CARTESIAN_POINT('Ctrl Pts',(34.177689437535,-0.250445930296054,23.0087857886416));
#39354=CARTESIAN_POINT('Ctrl Pts',(34.1465279851107,-0.204935197396313,
23.0056481306998));
#39355=CARTESIAN_POINT('Ctrl Pts',(34.1051820095339,-0.105164895936886,
23.0012239616958));
#39356=CARTESIAN_POINT('Ctrl Pts',(34.095,-0.0509015218992326,23.));
#39357=CARTESIAN_POINT('Ctrl Pts',(34.095,-5.55111512312578E-17,23.));
#39358=CARTESIAN_POINT('Ctrl Pts',(34.095,-6.93889390390723E-17,23.));
#39359=CARTESIAN_POINT('Ctrl Pts',(34.095,0.0509015218992325,23.));
#39360=CARTESIAN_POINT('Ctrl Pts',(34.1051820095339,0.105164895936886,23.0012239616958));
#39361=CARTESIAN_POINT('Ctrl Pts',(34.1465279851107,0.204935197396313,23.0056481306998));
#39362=CARTESIAN_POINT('Ctrl Pts',(34.177689437535,0.250445930296054,23.0087857886416));
#39363=CARTESIAN_POINT('Ctrl Pts',(34.2495542896821,0.322310782443173,23.0146857230619));
#39364=CARTESIAN_POINT('Ctrl Pts',(34.2950649266667,0.353472062708214,23.0178325988594));
#39365=CARTESIAN_POINT('Ctrl Pts',(34.3948349045423,0.39481791137655,23.0222778822844));
#39366=CARTESIAN_POINT('Ctrl Pts',(34.449098166481,0.405000000000001,23.0235111103298));
#39367=CARTESIAN_POINT('Ctrl Pts',(34.550901833519,0.405000000000001,23.0235111103298));
#39368=CARTESIAN_POINT('Ctrl Pts',(34.6051650954577,0.39481791137655,23.0222778822844));
#39369=CARTESIAN_POINT('Ctrl Pts',(34.7049350733333,0.353472062708214,23.0178325988594));
#39370=CARTESIAN_POINT('Ctrl Pts',(34.7504457103179,0.322310782443173,23.0146857230619));
#39371=CARTESIAN_POINT('Ctrl Pts',(34.822310562465,0.250445930296054,23.0087857886416));
#39372=CARTESIAN_POINT('Ctrl Pts',(34.8534720148893,0.204935197396313,23.0056481306998));
#39373=CARTESIAN_POINT('Ctrl Pts',(34.8948179904661,0.105164895936886,23.0012239616958));
#39374=CARTESIAN_POINT('Ctrl Pts',(34.905,0.0509015218992327,23.));
#39375=CARTESIAN_POINT('Ctrl Pts',(34.905,-0.0509015218992325,23.));
#39376=CARTESIAN_POINT('Ctrl Pts',(34.8948179904661,-0.105164895936886,
23.0012239616958));
#39377=CARTESIAN_POINT('Ctrl Pts',(34.8534720148893,-0.204935197396313,
23.0056481306998));
#39378=CARTESIAN_POINT('Ctrl Pts',(34.822310562465,-0.250445930296054,23.0087857886416));
#39379=CARTESIAN_POINT('Ctrl Pts',(34.7504457103179,-0.322310782443173,
23.0146857230619));
#39380=CARTESIAN_POINT('Ctrl Pts',(34.7049350733333,-0.353472062708218,
23.0178325988594));
#39381=CARTESIAN_POINT('Ctrl Pts',(34.6051650954577,-0.394817911376552,
23.0222778822844));
#39382=CARTESIAN_POINT('Ctrl Pts',(34.550901833519,-0.405000000000001,23.0235111103298));
#39383=CARTESIAN_POINT('Ctrl Pts',(34.5,-0.405000000000002,23.0235111103298));
#39384=CARTESIAN_POINT('Origin',(33.5,0.,30.4));
#39385=CARTESIAN_POINT('',(33.5,-1.005,29.8526071944086));
#39386=CARTESIAN_POINT('',(32.495,-2.14194167543114E-16,30.));
#39387=CARTESIAN_POINT('Ctrl Pts',(33.5,-1.005,29.8526071944086));
#39388=CARTESIAN_POINT('Ctrl Pts',(33.6269804671999,-1.005,29.8526071944086));
#39389=CARTESIAN_POINT('Ctrl Pts',(33.761899912268,-0.979475933914398,29.8605754646619));
#39390=CARTESIAN_POINT('Ctrl Pts',(34.0092777665881,-0.876698892882462,
29.8888404369081));
#39391=CARTESIAN_POINT('Ctrl Pts',(34.1218034634525,-0.799481166732521,
29.9086744581332));
#39392=CARTESIAN_POINT('Ctrl Pts',(34.2994591208888,-0.621825509296123,
29.9455131183184));
#39393=CARTESIAN_POINT('Ctrl Pts',(34.3766939521777,-0.509290792165725,
29.9649839652991));
#39394=CARTESIAN_POINT('Ctrl Pts',(34.479483580312,-0.261880374230206,29.9924074303405));
#39395=CARTESIAN_POINT('Ctrl Pts',(34.505,-0.126948956307063,30.));
#39396=CARTESIAN_POINT('Ctrl Pts',(34.505,0.126948956307063,30.));
#39397=CARTESIAN_POINT('Ctrl Pts',(34.479483580312,0.261880374230207,29.9924074303405));
#39398=CARTESIAN_POINT('Ctrl Pts',(34.3766939521777,0.509290792165726,29.9649839652991));
#39399=CARTESIAN_POINT('Ctrl Pts',(34.2994591208888,0.621825509296123,29.9455131183184));
#39400=CARTESIAN_POINT('Ctrl Pts',(34.1218034634525,0.799481166732521,29.9086744581332));
#39401=CARTESIAN_POINT('Ctrl Pts',(34.0092777665881,0.876698892882462,29.8888404369081));
#39402=CARTESIAN_POINT('Ctrl Pts',(33.761899912268,0.979475933914398,29.8605754646619));
#39403=CARTESIAN_POINT('Ctrl Pts',(33.6269804671999,1.005,29.8526071944086));
#39404=CARTESIAN_POINT('Ctrl Pts',(33.3730195328001,1.005,29.8526071944086));
#39405=CARTESIAN_POINT('Ctrl Pts',(33.238100087732,0.979475933914398,29.8605754646619));
#39406=CARTESIAN_POINT('Ctrl Pts',(32.9907222334119,0.876698892882462,29.8888404369081));
#39407=CARTESIAN_POINT('Ctrl Pts',(32.8781965365475,0.799481166732521,29.9086744581332));
#39408=CARTESIAN_POINT('Ctrl Pts',(32.7005408791112,0.621825509296124,29.9455131183184));
#39409=CARTESIAN_POINT('Ctrl Pts',(32.6233060478223,0.509290792165726,29.9649839652991));
#39410=CARTESIAN_POINT('Ctrl Pts',(32.520516419688,0.261880374230206,29.9924074303405));
#39411=CARTESIAN_POINT('Ctrl Pts',(32.495,0.126948956307063,30.));
#39412=CARTESIAN_POINT('Ctrl Pts',(32.495,3.88578058618805E-16,30.));
#39413=CARTESIAN_POINT('Ctrl Pts',(32.495,-2.4980018054066E-16,30.));
#39414=CARTESIAN_POINT('Ctrl Pts',(32.495,-0.126948956307063,30.));
#39415=CARTESIAN_POINT('Ctrl Pts',(32.520516419688,-0.261880374230207,29.9924074303405));
#39416=CARTESIAN_POINT('Ctrl Pts',(32.6233060478223,-0.509290792165726,
29.9649839652991));
#39417=CARTESIAN_POINT('Ctrl Pts',(32.7005408791112,-0.621825509296123,
29.9455131183184));
#39418=CARTESIAN_POINT('Ctrl Pts',(32.8781965365475,-0.799481166732521,
29.9086744581332));
#39419=CARTESIAN_POINT('Ctrl Pts',(32.9907222334119,-0.876698892882462,
29.8888404369081));
#39420=CARTESIAN_POINT('Ctrl Pts',(33.238100087732,-0.979475933914398,29.8605754646619));
#39421=CARTESIAN_POINT('Ctrl Pts',(33.3730195328001,-1.005,29.8526071944086));
#39422=CARTESIAN_POINT('Ctrl Pts',(33.5,-1.005,29.8526071944086));
#39423=CARTESIAN_POINT('',(32.495,-1.23077003314309E-16,31.8));
#39424=CARTESIAN_POINT('',(32.495,-1.23077003314309E-16,30.4));
#39425=CARTESIAN_POINT('Origin',(33.5,0.,31.8));
#39426=CARTESIAN_POINT('Origin',(34.105,0.,31.8));
#39427=CARTESIAN_POINT('',(32.895,-7.40911313484154E-17,31.8));
#39428=CARTESIAN_POINT('Origin',(33.5,0.,31.8));
#39429=CARTESIAN_POINT('Origin',(33.5,0.,32.65));
#39430=CARTESIAN_POINT('',(32.895,-7.40911313484154E-17,32.65));
#39431=CARTESIAN_POINT('Origin',(22.,0.,26.5));
#39432=CARTESIAN_POINT('',(8.,-3.5,26.5));
#39433=CARTESIAN_POINT('Origin',(8.,0.,26.5));
#39434=CARTESIAN_POINT('',(22.,-3.5,26.5));
#39435=CARTESIAN_POINT('Origin',(8.,5.5,26.5));
#76619=UNCERTAINTY_MEASURE_WITH_UNIT(LENGTH_MEASURE(0.001),#76661,
'DISTANCE_ACCURACY_VALUE',
'Maximum model space distance between geometric entities at asserted c
onnectivities');
#76638=UNCERTAINTY_MEASURE_WITH_UNIT(LENGTH_MEASURE(0.001),#76661,
'DISTANCE_ACCURACY_VALUE',
'Maximum model space distance between geometric entities at asserted c
onnectivities');
#76641=(
GEOMETRIC_REPRESENTATION_CONTEXT(3)
GLOBAL_UNCERTAINTY_ASSIGNED_CONTEXT((#76619))
GLOBAL_UNIT_ASSIGNED_CONTEXT((#76661,#76663,#76664))
REPRESENTATION_CONTEXT('','3D')
);
#76660=(
GEOMETRIC_REPRESENTATION_CONTEXT(3)
GLOBAL_UNCERTAINTY_ASSIGNED_CONTEXT((#76638))
GLOBAL_UNIT_ASSIGNED_CONTEXT((#76661,#76663,#76664))
REPRESENTATION_CONTEXT('','3D')
);
#76661=(
LENGTH_UNIT()
NAMED_UNIT(*)
SI_UNIT(.CENTI.,.METRE.)
);
#76663=(
NAMED_UNIT(*)
PLANE_ANGLE_UNIT()
SI_UNIT($,.RADIAN.)
);
#76664=(
NAMED_UNIT(*)
SI_UNIT($,.STERADIAN.)
SOLID_ANGLE_UNIT()
);
#76667=SHAPE_DEFINITION_REPRESENTATION(#76688,#76737);
#76688=PRODUCT_DEFINITION_SHAPE('',$,#76759);
#76737=SHAPE_REPRESENTATION('',(#27141),#76641);
#76756=PRODUCT_DEFINITION_CONTEXT('part definition',#76821,'design');
#76759=PRODUCT_DEFINITION('2026-10-26-11-12-31-151',
'02_Upper_Sliding_Tailstock_Casing',#76780,#76756);
#76780=PRODUCT_DEFINITION_FORMATION('',$,#76825);
#76821=APPLICATION_CONTEXT(
'Core Data for Automotive Mechanical Design Process');
#76822=PRODUCT_CONTEXT('part definition',#76821,'mechanical');
#76825=PRODUCT('2026-10-26-11-12-31-151',
'02_Upper_Sliding_Tailstock_Casing',$,(#76822));
#76886=COLOUR_RGB('Light Blue',0.38,0.62,0.78);
#76887=FILL_AREA_STYLE_COLOUR('',#76886);
#76888=FILL_AREA_STYLE('',(#76887));
#76889=SURFACE_STYLE_FILL_AREA(#76888);
#76890=SURFACE_SIDE_STYLE('',(#76889));
#76891=SURFACE_STYLE_USAGE(.BOTH.,#76890);
#76892=PRESENTATION_STYLE_ASSIGNMENT((#76891));
ENDSEC;
END-ISO-10303-21;
